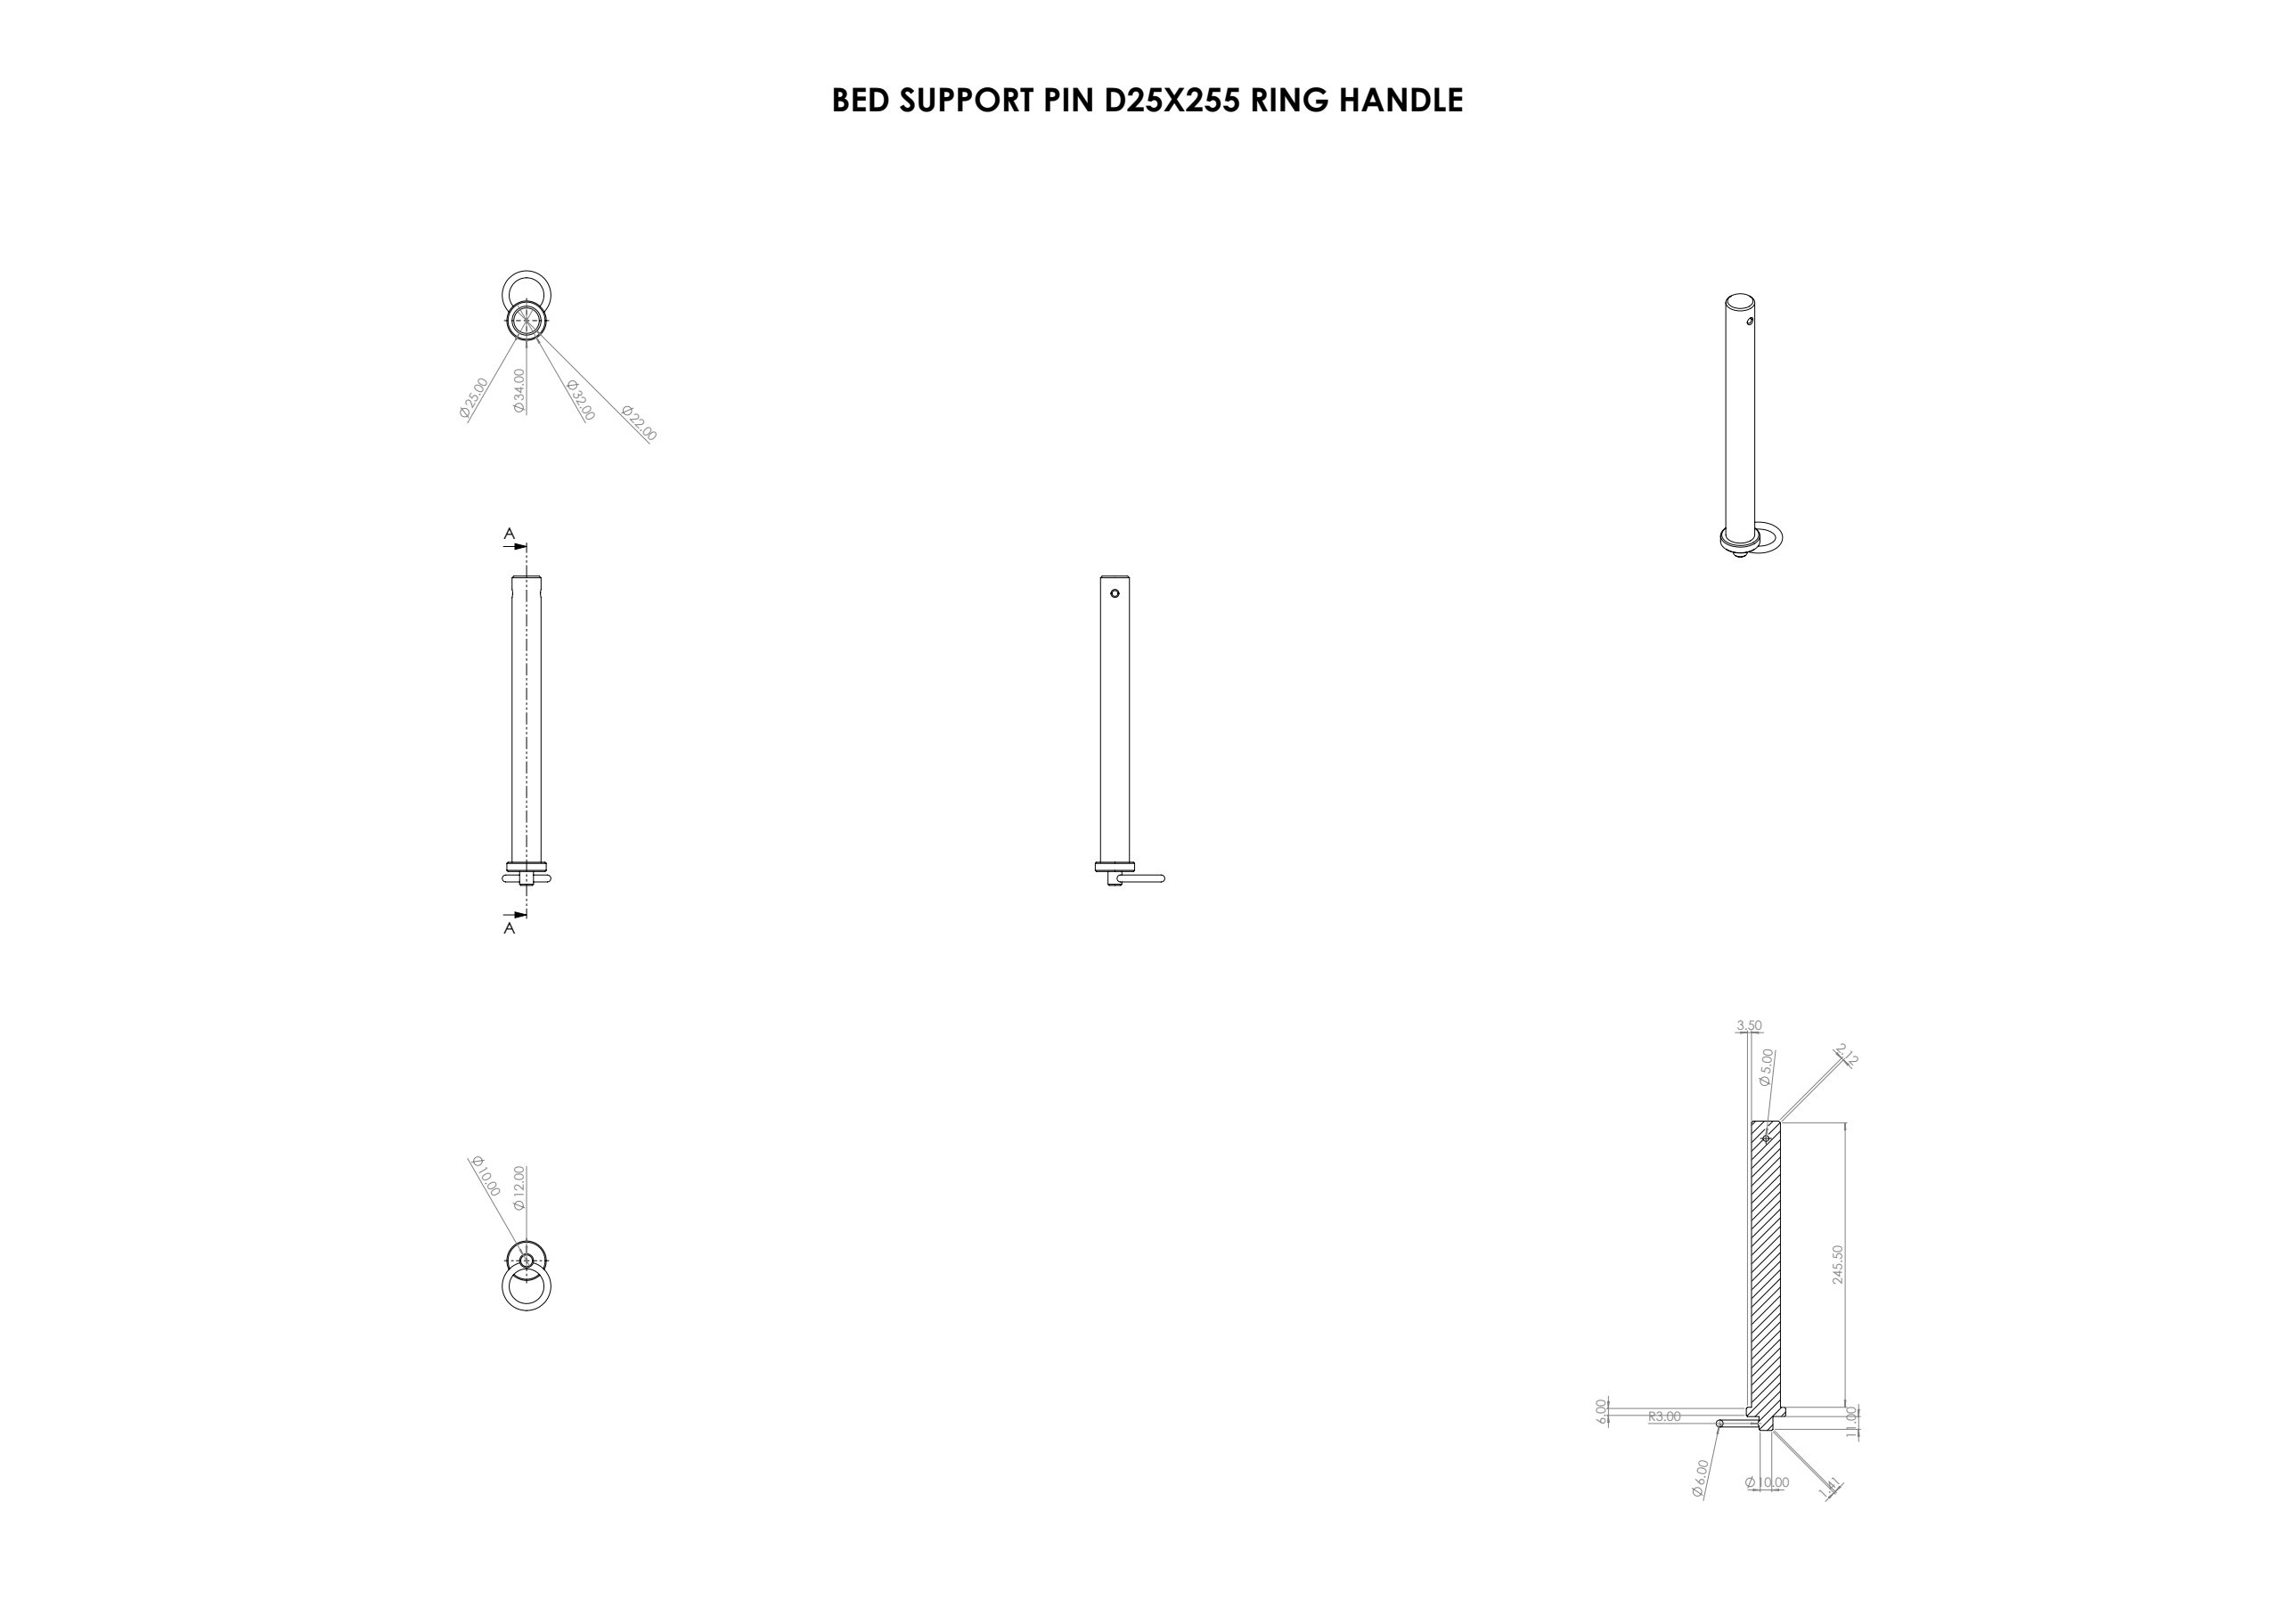
ISO-10303-21;
HEADER;
/* Generated by software containing ST-Developer
 * from STEP Tools, Inc. (www.steptools.com) 
 */

FILE_DESCRIPTION(
/* description */ (''),
/* implementation_level */ '2;1');

FILE_NAME(
/* name */ '05_Bed_Support_Pin_D25x255_Ring_Handle.step',
/* time_stamp */ '2026-10-20T10:03:03-07:00',
/* author */ (''),
/* organization */ (''),
/* preprocessor_version */ 'ST-DEVELOPER v20.2',
/* originating_system */ 'Autodesk Translation Framework v15.15.0.0',
/* authorisation */ '');

FILE_SCHEMA (('AUTOMOTIVE_DESIGN { 1 0 10303 214 3 1 1 }'));
ENDSEC;

DATA;
#10=MECHANICAL_DESIGN_GEOMETRIC_PRESENTATION_REPRESENTATION('',(#533),#71492);
#377=TOROIDAL_SURFACE('',#29987,1.8,0.299999999999997);
#390=SHAPE_REPRESENTATION_RELATIONSHIP('SRR','None',#71611,#409);
#409=ADVANCED_BREP_SHAPE_REPRESENTATION('',(#428),#71481);
#428=MANIFOLD_SOLID_BREP('Pin',#28467);
#533=STYLED_ITEM('',(#71887),#428);
#880=B_SPLINE_CURVE_WITH_KNOTS('',3,(#49263,#49264,#49265,#49266,#49267,
#49268,#49269,#49270,#49271,#49272,#49273,#49274,#49275,#49276,#49277,#49278,
#49279),.UNSPECIFIED.,.F.,.F.,(4,2,2,2,2,2,2,1,4),(0.,0.094448813972548,
0.188897627945096,0.283341149511147,0.377784671077197,0.472228192643248,
0.566671714209298,0.661120528181846,0.755569342154394),.UNSPECIFIED.);
#881=B_SPLINE_CURVE_WITH_KNOTS('',3,(#49280,#49281,#49282,#49283,#49284,
#49285,#49286,#49287,#49288,#49289,#49290,#49291,#49292,#49293,#49294,#49295,
#49296),.UNSPECIFIED.,.F.,.F.,(4,1,2,2,2,2,2,2,4),(0.755569342154394,0.850018156126942,
0.94446697009949,1.03891049166554,1.13335401323159,1.22779753479764,1.32224105636369,
1.41668987033624,1.51113868430879),.UNSPECIFIED.);
#882=B_SPLINE_CURVE_WITH_KNOTS('',3,(#49297,#49298,#49299,#49300,#49301,
#49302,#49303,#49304,#49305,#49306,#49307,#49308,#49309,#49310,#49311,#49312,
#49313,#49314,#49315,#49316,#49317,#49318,#49319,#49320,#49321,#49322,#49323,
#49324,#49325,#49326,#49327),.UNSPECIFIED.,.T.,.F.,(4,2,2,2,2,2,2,1,1,1,
2,2,2,2,2,2,4),(-1.51113868430879,-1.41668987033624,-1.32224105636369,-1.22779753479764,
-1.13335401323159,-1.03891049166554,-0.94446697009949,-0.850018156126942,
-0.755569342154394,-0.661120528181846,-0.566671714209298,-0.472228192643248,
-0.377784671077197,-0.283341149511147,-0.188897627945096,-0.094448813972548,
0.),.UNSPECIFIED.);
#883=B_SPLINE_CURVE_WITH_KNOTS('',3,(#49332,#49333,#49334,#49335,#49336,
#49337,#49338,#49339,#49340,#49341,#49342,#49343,#49344,#49345,#49346,#49347),
 .UNSPECIFIED.,.F.,.F.,(4,2,2,1,2,2,2,1,4),(0.,0.094448813972548,0.283341149511147,
0.330562910294172,0.377784671077197,0.472228192643248,0.566671714209298,
0.661120528181846,0.755569342154394),.UNSPECIFIED.);
#884=B_SPLINE_CURVE_WITH_KNOTS('',3,(#49348,#49349,#49350,#49351,#49352,
#49353,#49354,#49355,#49356,#49357,#49358,#49359,#49360,#49361,#49362,#49363,
#49364,#49365),.UNSPECIFIED.,.F.,.F.,(4,1,1,2,2,2,2,2,2,4),(0.755569342154394,
0.779181545647531,0.850018156126942,0.94446697009949,1.03891049166554,1.13335401323159,
1.22779753479764,1.32224105636369,1.41668987033624,1.51113868430879),
 .UNSPECIFIED.);
#885=B_SPLINE_CURVE_WITH_KNOTS('',3,(#49373,#49374,#49375,#49376,#49377,
#49378,#49379,#49380,#49381,#49382,#49383,#49384,#49385,#49386,#49387,#49388,
#49389,#49390,#49391,#49392,#49393,#49394,#49395,#49396,#49397,#49398,#49399,
#49400,#49401,#49402,#49403),.UNSPECIFIED.,.T.,.F.,(4,2,2,2,2,2,2,1,1,1,
1,2,2,2,1,2,2,4),(-1.51113868430879,-1.41668987033624,-1.32224105636369,
-1.22779753479764,-1.13335401323159,-1.03891049166554,-0.94446697009949,
-0.850018156126942,-0.779181545647531,-0.755569342154394,-0.661120528181846,
-0.566671714209298,-0.472228192643248,-0.377784671077197,-0.330562910294172,
-0.283341149511147,-0.094448813972548,0.),.UNSPECIFIED.);
#886=B_SPLINE_CURVE_WITH_KNOTS('',3,(#49535,#49536,#49537,#49538,#49539,
#49540,#49541,#49542),.UNSPECIFIED.,.F.,.F.,(4,2,2,4),(0.,0.128865571792524,
0.312353805988101,0.450725664145117),.UNSPECIFIED.);
#887=B_SPLINE_CURVE_WITH_KNOTS('',3,(#49544,#49545,#49546,#49547,#49548,
#49549,#49550,#49551,#49552,#49553,#49554,#49555,#49556,#49557,#49558,#49559,
#49560,#49561,#49562,#49563,#49564,#49565,#49566,#49567,#49568,#49569),
 .UNSPECIFIED.,.F.,.F.,(4,2,2,2,2,2,2,2,2,2,2,2,4),(3.03100409690103,3.10724965658915,
3.31962805616212,3.55816001091835,3.71946361604111,3.8667157448743,4.00577882547157,
4.14436012284324,4.2798687704017,4.40986006512752,4.53061941509967,4.63980546599939,
4.72630087619969),.UNSPECIFIED.);
#888=B_SPLINE_CURVE_WITH_KNOTS('',3,(#49570,#49571,#49572,#49573,#49574,
#49575,#49576,#49577,#49578,#49579,#49580,#49581,#49582,#49583,#49584,#49585,
#49586,#49587,#49588,#49589,#49590,#49591,#49592,#49593,#49594,#49595,#49596,
#49597,#49598,#49599,#49600,#49601),.UNSPECIFIED.,.F.,.F.,(4,2,2,2,2,2,
2,2,2,2,2,2,2,2,2,4),(0.450725664145117,0.504434541071938,0.741766796410238,
1.06081742489875,1.26362192220824,1.44561364264116,1.61660881920843,1.78645082881554,
1.9531313289519,2.11323423539159,2.26278985619793,2.3977184604128,2.53060287457306,
2.68742490157839,2.91311758246269,3.03100409690103),.UNSPECIFIED.);
#1458=B_SPLINE_SURFACE_WITH_KNOTS('',3,3,((#49135,#49136,#49137,#49138,
#49139,#49140,#49141,#49142,#49143,#49144,#49145,#49146,#49147,#49148,#49149,
#49150,#49151,#49152,#49153,#49154,#49155,#49156,#49157,#49158,#49159,#49160,
#49161,#49162,#49163,#49164,#49165),(#49166,#49167,#49168,#49169,#49170,
#49171,#49172,#49173,#49174,#49175,#49176,#49177,#49178,#49179,#49180,#49181,
#49182,#49183,#49184,#49185,#49186,#49187,#49188,#49189,#49190,#49191,#49192,
#49193,#49194,#49195,#49196),(#49197,#49198,#49199,#49200,#49201,#49202,
#49203,#49204,#49205,#49206,#49207,#49208,#49209,#49210,#49211,#49212,#49213,
#49214,#49215,#49216,#49217,#49218,#49219,#49220,#49221,#49222,#49223,#49224,
#49225,#49226,#49227),(#49228,#49229,#49230,#49231,#49232,#49233,#49234,
#49235,#49236,#49237,#49238,#49239,#49240,#49241,#49242,#49243,#49244,#49245,
#49246,#49247,#49248,#49249,#49250,#49251,#49252,#49253,#49254,#49255,#49256,
#49257,#49258)),.UNSPECIFIED.,.F.,.T.,.F.,(4,4),(4,2,2,2,2,2,2,1,1,1,2,
2,2,2,2,2,4),(0.,1.),(0.,0.094448813972548,0.188897627945096,0.283341149511147,
0.377784671077197,0.472228192643248,0.566671714209298,0.661120528181846,
0.755569342154394,0.850018156126942,0.94446697009949,1.03891049166554,1.13335401323159,
1.22779753479764,1.32224105636369,1.41668987033624,1.51113868430879),
 .UNSPECIFIED.);
#1459=B_SPLINE_SURFACE_WITH_KNOTS('',3,3,((#49404,#49405,#49406,#49407,
#49408,#49409,#49410,#49411,#49412,#49413,#49414,#49415,#49416,#49417,#49418,
#49419,#49420,#49421,#49422,#49423,#49424,#49425,#49426,#49427,#49428,#49429,
#49430,#49431,#49432,#49433,#49434),(#49435,#49436,#49437,#49438,#49439,
#49440,#49441,#49442,#49443,#49444,#49445,#49446,#49447,#49448,#49449,#49450,
#49451,#49452,#49453,#49454,#49455,#49456,#49457,#49458,#49459,#49460,#49461,
#49462,#49463,#49464,#49465),(#49466,#49467,#49468,#49469,#49470,#49471,
#49472,#49473,#49474,#49475,#49476,#49477,#49478,#49479,#49480,#49481,#49482,
#49483,#49484,#49485,#49486,#49487,#49488,#49489,#49490,#49491,#49492,#49493,
#49494,#49495,#49496),(#49497,#49498,#49499,#49500,#49501,#49502,#49503,
#49504,#49505,#49506,#49507,#49508,#49509,#49510,#49511,#49512,#49513,#49514,
#49515,#49516,#49517,#49518,#49519,#49520,#49521,#49522,#49523,#49524,#49525,
#49526,#49527)),.UNSPECIFIED.,.F.,.T.,.F.,(4,4),(4,2,2,1,2,2,2,1,1,1,1,
2,2,2,2,2,2,4),(0.,1.),(0.,0.094448813972548,0.283341149511147,0.330562910294172,
0.377784671077197,0.472228192643248,0.566671714209298,0.661120528181846,
0.755569342154394,0.779181545647531,0.850018156126942,0.94446697009949,
1.03891049166554,1.13335401323159,1.22779753479764,1.32224105636369,1.41668987033624,
1.51113868430879),.UNSPECIFIED.);
#1668=CYLINDRICAL_SURFACE('',#29983,0.25);
#1669=CYLINDRICAL_SURFACE('',#29984,1.25);
#1670=CYLINDRICAL_SURFACE('',#29990,0.599999999999994);
#1671=CYLINDRICAL_SURFACE('',#30000,1.7);
#1948=FACE_BOUND('',#5603,.T.);
#1949=FACE_BOUND('',#5604,.T.);
#1950=FACE_BOUND('',#5607,.T.);
#1951=FACE_BOUND('',#5612,.T.);
#1952=FACE_BOUND('',#5617,.T.);
#2465=CIRCLE('',#29985,1.25);
#2466=CIRCLE('',#29986,1.25);
#2467=CIRCLE('',#29988,0.299999999999997);
#2468=CIRCLE('',#29989,1.5);
#2469=CIRCLE('',#29991,0.599999999999994);
#2470=CIRCLE('',#29992,0.599999999999994);
#2471=CIRCLE('',#29994,0.5);
#2472=CIRCLE('',#29997,1.59999999999999);
#2473=CIRCLE('',#29999,1.7);
#2474=CIRCLE('',#30001,1.7);
#2475=CIRCLE('',#30003,1.59999999999999);
#2476=CIRCLE('',#30006,1.09999999999999);
#2861=CONICAL_SURFACE('',#29995,0.549999999999997,0.785398163397422);
#2862=CONICAL_SURFACE('',#29998,1.65000000000001,0.785398163397493);
#2863=CONICAL_SURFACE('',#30002,1.65000000000001,0.785398163397484);
#2864=CONICAL_SURFACE('',#30005,1.175,0.785398163397466);
#3946=FACE_OUTER_BOUND('',#5600,.T.);
#3947=FACE_OUTER_BOUND('',#5601,.T.);
#3948=FACE_OUTER_BOUND('',#5602,.T.);
#3949=FACE_OUTER_BOUND('',#5605,.T.);
#3950=FACE_OUTER_BOUND('',#5606,.T.);
#3951=FACE_OUTER_BOUND('',#5608,.T.);
#3952=FACE_OUTER_BOUND('',#5609,.T.);
#3953=FACE_OUTER_BOUND('',#5610,.T.);
#3954=FACE_OUTER_BOUND('',#5611,.T.);
#3955=FACE_OUTER_BOUND('',#5613,.T.);
#3956=FACE_OUTER_BOUND('',#5614,.T.);
#3957=FACE_OUTER_BOUND('',#5615,.T.);
#3958=FACE_OUTER_BOUND('',#5616,.T.);
#3959=FACE_OUTER_BOUND('',#5618,.T.);
#3960=FACE_OUTER_BOUND('',#5619,.T.);
#5600=EDGE_LOOP('',(#22975,#22976,#22977,#22978,#22979));
#5601=EDGE_LOOP('',(#22980,#22981,#22982,#22983,#22984,#22985));
#5602=EDGE_LOOP('',(#22986,#22987,#22988,#22989));
#5603=EDGE_LOOP('',(#22990));
#5604=EDGE_LOOP('',(#22991));
#5605=EDGE_LOOP('',(#22992,#22993,#22994,#22995,#22996));
#5606=EDGE_LOOP('',(#22997,#22998,#22999,#23000));
#5607=EDGE_LOOP('',(#23001,#23002,#23003));
#5608=EDGE_LOOP('',(#23004,#23005,#23006,#23007,#23008,#23009,#23010,#23011,
#23012));
#5609=EDGE_LOOP('',(#23013));
#5610=EDGE_LOOP('',(#23014,#23015,#23016,#23017));
#5611=EDGE_LOOP('',(#23018));
#5612=EDGE_LOOP('',(#23019));
#5613=EDGE_LOOP('',(#23020,#23021,#23022,#23023));
#5614=EDGE_LOOP('',(#23024,#23025,#23026,#23027));
#5615=EDGE_LOOP('',(#23028,#23029,#23030,#23031));
#5616=EDGE_LOOP('',(#23032));
#5617=EDGE_LOOP('',(#23033));
#5618=EDGE_LOOP('',(#23034,#23035,#23036,#23037));
#5619=EDGE_LOOP('',(#23038));
#7997=LINE('',#49261,#10485);
#7998=LINE('',#49330,#10486);
#7999=LINE('',#49370,#10487);
#8000=LINE('',#49528,#10488);
#8001=LINE('',#49605,#10489);
#8002=LINE('',#49607,#10490);
#8003=LINE('',#49613,#10491);
#8004=LINE('',#49620,#10492);
#8005=LINE('',#49624,#10493);
#8006=LINE('',#49628,#10494);
#8007=LINE('',#49633,#10495);
#10485=VECTOR('',#35140,1.);
#10486=VECTOR('',#35143,0.25);
#10487=VECTOR('',#35148,1.25);
#10488=VECTOR('',#35151,1.);
#10489=VECTOR('',#35162,0.599999999999994);
#10490=VECTOR('',#35163,0.599999999999994);
#10491=VECTOR('',#35172,0.549999999999997);
#10492=VECTOR('',#35181,1.65000000000001);
#10493=VECTOR('',#35186,1.7);
#10494=VECTOR('',#35191,1.65000000000001);
#10495=VECTOR('',#35198,1.175);
#12863=VERTEX_POINT('',#49259);
#12864=VERTEX_POINT('',#49260);
#12865=VERTEX_POINT('',#49262);
#12866=VERTEX_POINT('',#49329);
#12867=VERTEX_POINT('',#49331);
#12868=VERTEX_POINT('',#49367);
#12869=VERTEX_POINT('',#49369);
#12870=VERTEX_POINT('',#49372);
#12871=VERTEX_POINT('',#49530);
#12872=VERTEX_POINT('',#49533);
#12873=VERTEX_POINT('',#49534);
#12874=VERTEX_POINT('',#49543);
#12875=VERTEX_POINT('',#49603);
#12876=VERTEX_POINT('',#49606);
#12877=VERTEX_POINT('',#49610);
#12878=VERTEX_POINT('',#49615);
#12879=VERTEX_POINT('',#49618);
#12880=VERTEX_POINT('',#49622);
#12881=VERTEX_POINT('',#49626);
#12882=VERTEX_POINT('',#49631);
#16371=EDGE_CURVE('',#12863,#12864,#7997,.T.);
#16372=EDGE_CURVE('',#12864,#12865,#880,.T.);
#16373=EDGE_CURVE('',#12865,#12864,#881,.T.);
#16374=EDGE_CURVE('',#12863,#12863,#882,.T.);
#16375=EDGE_CURVE('',#12865,#12866,#7998,.T.);
#16376=EDGE_CURVE('',#12867,#12866,#883,.T.);
#16377=EDGE_CURVE('',#12866,#12867,#884,.T.);
#16378=EDGE_CURVE('',#12868,#12868,#2465,.T.);
#16379=EDGE_CURVE('',#12868,#12869,#7999,.T.);
#16380=EDGE_CURVE('',#12869,#12869,#2466,.T.);
#16381=EDGE_CURVE('',#12870,#12870,#885,.T.);
#16382=EDGE_CURVE('',#12870,#12867,#8000,.T.);
#16383=EDGE_CURVE('',#12871,#12871,#2467,.T.);
#16384=EDGE_CURVE('',#12871,#12871,#2468,.T.);
#16385=EDGE_CURVE('',#12872,#12873,#886,.T.);
#16386=EDGE_CURVE('',#12874,#12872,#887,.T.);
#16387=EDGE_CURVE('',#12873,#12874,#888,.T.);
#16388=EDGE_CURVE('',#12875,#12875,#2469,.T.);
#16389=EDGE_CURVE('',#12875,#12874,#8001,.T.);
#16390=EDGE_CURVE('',#12873,#12876,#8002,.T.);
#16391=EDGE_CURVE('',#12876,#12876,#2470,.T.);
#16392=EDGE_CURVE('',#12877,#12877,#2471,.T.);
#16393=EDGE_CURVE('',#12876,#12877,#8003,.T.);
#16394=EDGE_CURVE('',#12878,#12878,#2472,.T.);
#16395=EDGE_CURVE('',#12879,#12879,#2473,.T.);
#16396=EDGE_CURVE('',#12879,#12878,#8004,.T.);
#16397=EDGE_CURVE('',#12880,#12880,#2474,.T.);
#16398=EDGE_CURVE('',#12880,#12879,#8005,.T.);
#16399=EDGE_CURVE('',#12881,#12881,#2475,.T.);
#16400=EDGE_CURVE('',#12881,#12880,#8006,.T.);
#16401=EDGE_CURVE('',#12882,#12882,#2476,.T.);
#16402=EDGE_CURVE('',#12882,#12868,#8007,.T.);
#22975=ORIENTED_EDGE('',*,*,#16371,.T.);
#22976=ORIENTED_EDGE('',*,*,#16372,.T.);
#22977=ORIENTED_EDGE('',*,*,#16373,.T.);
#22978=ORIENTED_EDGE('',*,*,#16371,.F.);
#22979=ORIENTED_EDGE('',*,*,#16374,.T.);
#22980=ORIENTED_EDGE('',*,*,#16372,.F.);
#22981=ORIENTED_EDGE('',*,*,#16373,.F.);
#22982=ORIENTED_EDGE('',*,*,#16375,.T.);
#22983=ORIENTED_EDGE('',*,*,#16376,.F.);
#22984=ORIENTED_EDGE('',*,*,#16377,.F.);
#22985=ORIENTED_EDGE('',*,*,#16375,.F.);
#22986=ORIENTED_EDGE('',*,*,#16378,.F.);
#22987=ORIENTED_EDGE('',*,*,#16379,.T.);
#22988=ORIENTED_EDGE('',*,*,#16380,.T.);
#22989=ORIENTED_EDGE('',*,*,#16379,.F.);
#22990=ORIENTED_EDGE('',*,*,#16381,.F.);
#22991=ORIENTED_EDGE('',*,*,#16374,.F.);
#22992=ORIENTED_EDGE('',*,*,#16382,.T.);
#22993=ORIENTED_EDGE('',*,*,#16376,.T.);
#22994=ORIENTED_EDGE('',*,*,#16377,.T.);
#22995=ORIENTED_EDGE('',*,*,#16382,.F.);
#22996=ORIENTED_EDGE('',*,*,#16381,.T.);
#22997=ORIENTED_EDGE('',*,*,#16383,.F.);
#22998=ORIENTED_EDGE('',*,*,#16384,.T.);
#22999=ORIENTED_EDGE('',*,*,#16383,.T.);
#23000=ORIENTED_EDGE('',*,*,#16384,.F.);
#23001=ORIENTED_EDGE('',*,*,#16385,.F.);
#23002=ORIENTED_EDGE('',*,*,#16386,.F.);
#23003=ORIENTED_EDGE('',*,*,#16387,.F.);
#23004=ORIENTED_EDGE('',*,*,#16388,.F.);
#23005=ORIENTED_EDGE('',*,*,#16389,.T.);
#23006=ORIENTED_EDGE('',*,*,#16386,.T.);
#23007=ORIENTED_EDGE('',*,*,#16385,.T.);
#23008=ORIENTED_EDGE('',*,*,#16390,.T.);
#23009=ORIENTED_EDGE('',*,*,#16391,.T.);
#23010=ORIENTED_EDGE('',*,*,#16390,.F.);
#23011=ORIENTED_EDGE('',*,*,#16387,.T.);
#23012=ORIENTED_EDGE('',*,*,#16389,.F.);
#23013=ORIENTED_EDGE('',*,*,#16392,.F.);
#23014=ORIENTED_EDGE('',*,*,#16391,.F.);
#23015=ORIENTED_EDGE('',*,*,#16393,.T.);
#23016=ORIENTED_EDGE('',*,*,#16392,.T.);
#23017=ORIENTED_EDGE('',*,*,#16393,.F.);
#23018=ORIENTED_EDGE('',*,*,#16394,.F.);
#23019=ORIENTED_EDGE('',*,*,#16388,.T.);
#23020=ORIENTED_EDGE('',*,*,#16395,.F.);
#23021=ORIENTED_EDGE('',*,*,#16396,.T.);
#23022=ORIENTED_EDGE('',*,*,#16394,.T.);
#23023=ORIENTED_EDGE('',*,*,#16396,.F.);
#23024=ORIENTED_EDGE('',*,*,#16397,.F.);
#23025=ORIENTED_EDGE('',*,*,#16398,.T.);
#23026=ORIENTED_EDGE('',*,*,#16395,.T.);
#23027=ORIENTED_EDGE('',*,*,#16398,.F.);
#23028=ORIENTED_EDGE('',*,*,#16399,.F.);
#23029=ORIENTED_EDGE('',*,*,#16400,.T.);
#23030=ORIENTED_EDGE('',*,*,#16397,.T.);
#23031=ORIENTED_EDGE('',*,*,#16400,.F.);
#23032=ORIENTED_EDGE('',*,*,#16399,.T.);
#23033=ORIENTED_EDGE('',*,*,#16380,.F.);
#23034=ORIENTED_EDGE('',*,*,#16401,.F.);
#23035=ORIENTED_EDGE('',*,*,#16402,.T.);
#23036=ORIENTED_EDGE('',*,*,#16378,.T.);
#23037=ORIENTED_EDGE('',*,*,#16402,.F.);
#23038=ORIENTED_EDGE('',*,*,#16401,.T.);
#26669=PLANE('',#29993);
#26670=PLANE('',#29996);
#26671=PLANE('',#30004);
#26672=PLANE('',#30007);
#27854=ADVANCED_FACE('',(#3946),#1458,.T.);
#27855=ADVANCED_FACE('',(#3947),#1668,.F.);
#27856=ADVANCED_FACE('',(#3948,#1948,#1949),#1669,.T.);
#27857=ADVANCED_FACE('',(#3949),#1459,.T.);
#27858=ADVANCED_FACE('',(#3950,#1950),#377,.T.);
#27859=ADVANCED_FACE('',(#3951),#1670,.T.);
#27860=ADVANCED_FACE('',(#3952),#26669,.T.);
#27861=ADVANCED_FACE('',(#3953),#2861,.T.);
#27862=ADVANCED_FACE('',(#3954,#1951),#26670,.T.);
#27863=ADVANCED_FACE('',(#3955),#2862,.T.);
#27864=ADVANCED_FACE('',(#3956),#1671,.T.);
#27865=ADVANCED_FACE('',(#3957),#2863,.T.);
#27866=ADVANCED_FACE('',(#3958,#1952),#26671,.T.);
#27867=ADVANCED_FACE('',(#3959),#2864,.T.);
#27868=ADVANCED_FACE('',(#3960),#26672,.T.);
#28467=CLOSED_SHELL('',(#27854,#27855,#27856,#27857,#27858,#27859,#27860,
#27861,#27862,#27863,#27864,#27865,#27866,#27867,#27868));
#29982=AXIS2_PLACEMENT_3D('',#49134,#35138,#35139);
#29983=AXIS2_PLACEMENT_3D('',#49328,#35141,#35142);
#29984=AXIS2_PLACEMENT_3D('',#49366,#35144,#35145);
#29985=AXIS2_PLACEMENT_3D('',#49368,#35146,#35147);
#29986=AXIS2_PLACEMENT_3D('',#49371,#35149,#35150);
#29987=AXIS2_PLACEMENT_3D('',#49529,#35152,#35153);
#29988=AXIS2_PLACEMENT_3D('',#49531,#35154,#35155);
#29989=AXIS2_PLACEMENT_3D('',#49532,#35156,#35157);
#29990=AXIS2_PLACEMENT_3D('',#49602,#35158,#35159);
#29991=AXIS2_PLACEMENT_3D('',#49604,#35160,#35161);
#29992=AXIS2_PLACEMENT_3D('',#49608,#35164,#35165);
#29993=AXIS2_PLACEMENT_3D('',#49609,#35166,#35167);
#29994=AXIS2_PLACEMENT_3D('',#49611,#35168,#35169);
#29995=AXIS2_PLACEMENT_3D('',#49612,#35170,#35171);
#29996=AXIS2_PLACEMENT_3D('',#49614,#35173,#35174);
#29997=AXIS2_PLACEMENT_3D('',#49616,#35175,#35176);
#29998=AXIS2_PLACEMENT_3D('',#49617,#35177,#35178);
#29999=AXIS2_PLACEMENT_3D('',#49619,#35179,#35180);
#30000=AXIS2_PLACEMENT_3D('',#49621,#35182,#35183);
#30001=AXIS2_PLACEMENT_3D('',#49623,#35184,#35185);
#30002=AXIS2_PLACEMENT_3D('',#49625,#35187,#35188);
#30003=AXIS2_PLACEMENT_3D('',#49627,#35189,#35190);
#30004=AXIS2_PLACEMENT_3D('',#49629,#35192,#35193);
#30005=AXIS2_PLACEMENT_3D('',#49630,#35194,#35195);
#30006=AXIS2_PLACEMENT_3D('',#49632,#35196,#35197);
#30007=AXIS2_PLACEMENT_3D('',#49634,#35199,#35200);
#35138=DIRECTION('axis',(0.,0.,1.));
#35139=DIRECTION('refdir',(1.,0.,0.));
#35140=DIRECTION('',(0.616833943686132,1.43989874226525E-14,0.787093314618168));
#35141=DIRECTION('center_axis',(1.,0.,0.));
#35142=DIRECTION('ref_axis',(0.,0.,-1.));
#35143=DIRECTION('',(1.,0.,0.));
#35144=DIRECTION('center_axis',(0.,1.,0.));
#35145=DIRECTION('ref_axis',(0.,0.,1.));
#35146=DIRECTION('center_axis',(0.,1.,0.));
#35147=DIRECTION('ref_axis',(1.,0.,0.));
#35148=DIRECTION('',(0.,-1.,0.));
#35149=DIRECTION('center_axis',(0.,1.,0.));
#35150=DIRECTION('ref_axis',(1.,0.,0.));
#35151=DIRECTION('',(-0.616833943686132,0.,0.787093314618168));
#35152=DIRECTION('center_axis',(0.,1.,0.));
#35153=DIRECTION('ref_axis',(0.,0.,1.));
#35154=DIRECTION('center_axis',(-1.,0.,0.));
#35155=DIRECTION('ref_axis',(0.,0.,-1.));
#35156=DIRECTION('center_axis',(0.,-1.,0.));
#35157=DIRECTION('ref_axis',(0.,0.,1.));
#35158=DIRECTION('center_axis',(0.,1.,0.));
#35159=DIRECTION('ref_axis',(0.,0.,1.));
#35160=DIRECTION('center_axis',(0.,1.,0.));
#35161=DIRECTION('ref_axis',(0.,0.,1.));
#35162=DIRECTION('',(0.,-1.,0.));
#35163=DIRECTION('',(0.,-1.,0.));
#35164=DIRECTION('center_axis',(0.,1.,0.));
#35165=DIRECTION('ref_axis',(1.,0.,0.));
#35166=DIRECTION('center_axis',(0.,-1.,0.));
#35167=DIRECTION('ref_axis',(0.,0.,-1.));
#35168=DIRECTION('center_axis',(0.,1.,0.));
#35169=DIRECTION('ref_axis',(1.,0.,0.));
#35170=DIRECTION('center_axis',(0.,1.,0.));
#35171=DIRECTION('ref_axis',(0.,0.,1.));
#35172=DIRECTION('',(8.6595605623547E-17,-0.707106781186566,0.707106781186529));
#35173=DIRECTION('center_axis',(0.,-1.,0.));
#35174=DIRECTION('ref_axis',(0.,0.,-1.));
#35175=DIRECTION('center_axis',(0.,1.,0.));
#35176=DIRECTION('ref_axis',(1.,0.,0.));
#35177=DIRECTION('center_axis',(0.,1.,0.));
#35178=DIRECTION('ref_axis',(0.,0.,1.));
#35179=DIRECTION('center_axis',(0.,1.,0.));
#35180=DIRECTION('ref_axis',(1.,0.,0.));
#35181=DIRECTION('',(8.65956056235532E-17,-0.707106781186516,0.707106781186579));
#35182=DIRECTION('center_axis',(0.,1.,0.));
#35183=DIRECTION('ref_axis',(0.,0.,1.));
#35184=DIRECTION('center_axis',(0.,1.,0.));
#35185=DIRECTION('ref_axis',(1.,0.,0.));
#35186=DIRECTION('',(0.,-1.,0.));
#35187=DIRECTION('center_axis',(0.,-1.,0.));
#35188=DIRECTION('ref_axis',(0.,0.,1.));
#35189=DIRECTION('center_axis',(0.,1.,0.));
#35190=DIRECTION('ref_axis',(1.,0.,0.));
#35191=DIRECTION('',(-8.65956056235524E-17,-0.707106781186522,-0.707106781186573));
#35192=DIRECTION('center_axis',(0.,1.,0.));
#35193=DIRECTION('ref_axis',(0.,0.,1.));
#35194=DIRECTION('center_axis',(0.,-1.,0.));
#35195=DIRECTION('ref_axis',(0.,0.,1.));
#35196=DIRECTION('center_axis',(0.,1.,0.));
#35197=DIRECTION('ref_axis',(1.,0.,0.));
#35198=DIRECTION('',(-8.65956056235509E-17,-0.707106781186535,-0.70710678118656));
#35199=DIRECTION('center_axis',(0.,1.,0.));
#35200=DIRECTION('ref_axis',(0.,0.,1.));
#49134=CARTESIAN_POINT('',(0.,0.,0.));
#49135=CARTESIAN_POINT('Ctrl Pts',(28.7991583057917,11.,74.402898825339));
#49136=CARTESIAN_POINT('Ctrl Pts',(28.7991583057917,11.0443255072037,74.402898825339));
#49137=CARTESIAN_POINT('Ctrl Pts',(28.7965453592084,11.0915510411579,74.4116063134345));
#49138=CARTESIAN_POINT('Ctrl Pts',(28.7871669871617,11.1779078402817,74.4468238161368));
#49139=CARTESIAN_POINT('Ctrl Pts',(28.7806043669257,11.2170846527409,74.4732883033298));
#49140=CARTESIAN_POINT('Ctrl Pts',(28.7683045654192,11.2788962751735,74.5344620266402));
#49141=CARTESIAN_POINT('Ctrl Pts',(28.7617930434695,11.3057060685816,74.5732868944695));
#49142=CARTESIAN_POINT('Ctrl Pts',(28.7525231854577,11.3414465815878,74.65904064169));
#49143=CARTESIAN_POINT('Ctrl Pts',(28.7499823739105,11.3502679248349,74.7059347785805));
#49144=CARTESIAN_POINT('Ctrl Pts',(28.7499717367413,11.3503212800739,74.7941254313177));
#49145=CARTESIAN_POINT('Ctrl Pts',(28.7525477553864,11.3414466364947,74.8410052800481));
#49146=CARTESIAN_POINT('Ctrl Pts',(28.7618133828337,11.3058394721478,74.9267618361903));
#49147=CARTESIAN_POINT('Ctrl Pts',(28.7683297787118,11.2789656668451,74.9656153280843));
#49148=CARTESIAN_POINT('Ctrl Pts',(28.7806136472154,11.2174765285995,75.0267085651774));
#49149=CARTESIAN_POINT('Ctrl Pts',(28.7938779355307,11.137485266407,75.079826557824));
#49150=CARTESIAN_POINT('Ctrl Pts',(28.8019055096204,11.,75.1059958179575));
#49151=CARTESIAN_POINT('Ctrl Pts',(28.7938779355307,10.8625147335932,75.079826557824));
#49152=CARTESIAN_POINT('Ctrl Pts',(28.7806136472154,10.7825234714004,75.0267085651771));
#49153=CARTESIAN_POINT('Ctrl Pts',(28.7683297787118,10.7210343331551,74.9656153280842));
#49154=CARTESIAN_POINT('Ctrl Pts',(28.7618133828337,10.6941605278523,74.9267618361901));
#49155=CARTESIAN_POINT('Ctrl Pts',(28.7525477553864,10.6585533635054,74.8410052800478));
#49156=CARTESIAN_POINT('Ctrl Pts',(28.7499717367413,10.6496787199262,74.7941254313175));
#49157=CARTESIAN_POINT('Ctrl Pts',(28.7499823739105,10.6497320751652,74.7059347785801));
#49158=CARTESIAN_POINT('Ctrl Pts',(28.7525231854577,10.6585534184123,74.6590406416897));
#49159=CARTESIAN_POINT('Ctrl Pts',(28.7617930434695,10.6942939314186,74.5732868944692));
#49160=CARTESIAN_POINT('Ctrl Pts',(28.7683045654192,10.7211037248264,74.5344620266403));
#49161=CARTESIAN_POINT('Ctrl Pts',(28.7806043669256,10.7829153472589,74.4732883033299));
#49162=CARTESIAN_POINT('Ctrl Pts',(28.7871669871616,10.8220921597181,74.4468238161368));
#49163=CARTESIAN_POINT('Ctrl Pts',(28.7965453592083,10.9084489588421,74.4116063134345));
#49164=CARTESIAN_POINT('Ctrl Pts',(28.7991583057917,10.9556744927962,74.402898825339));
#49165=CARTESIAN_POINT('Ctrl Pts',(28.7991583057917,11.,74.402898825339));
#49166=CARTESIAN_POINT('Ctrl Pts',(28.8245239133973,11.,74.4352658835594));
#49167=CARTESIAN_POINT('Ctrl Pts',(28.8245139996716,11.0409058476698,74.4352690808426));
#49168=CARTESIAN_POINT('Ctrl Pts',(28.8222946915156,11.0844693260521,74.4435587606527));
#49169=CARTESIAN_POINT('Ctrl Pts',(28.8143446526051,11.1634798118501,74.4766846891437));
#49170=CARTESIAN_POINT('Ctrl Pts',(28.8088018057836,11.1989487338351,74.5013491133979));
#49171=CARTESIAN_POINT('Ctrl Pts',(28.7984971202627,11.2543047022451,74.5574809291687));
#49172=CARTESIAN_POINT('Ctrl Pts',(28.7930705898665,11.277994263562,74.5926796862592));
#49173=CARTESIAN_POINT('Ctrl Pts',(28.7854083939203,11.3092896913271,74.6694190769384));
#49174=CARTESIAN_POINT('Ctrl Pts',(28.783317023756,11.316933318266,74.7109865811412));
#49175=CARTESIAN_POINT('Ctrl Pts',(28.7833092717601,11.3169759220082,74.789072841938));
#49176=CARTESIAN_POINT('Ctrl Pts',(28.7854300007706,11.3093021925761,74.8306284308288));
#49177=CARTESIAN_POINT('Ctrl Pts',(28.7930936893998,11.2781129419873,74.9073660164418));
#49178=CARTESIAN_POINT('Ctrl Pts',(28.7985190764957,11.2543992363159,74.9426040045736));
#49179=CARTESIAN_POINT('Ctrl Pts',(28.8088155168561,11.1992993473659,74.998632839126));
#49180=CARTESIAN_POINT('Ctrl Pts',(28.8200190370477,11.1268998693587,75.0482404349203));
#49181=CARTESIAN_POINT('Ctrl Pts',(28.8268763497815,11.,75.0732472458756));
#49182=CARTESIAN_POINT('Ctrl Pts',(28.8200190370477,10.8731001306415,75.0482404349203));
#49183=CARTESIAN_POINT('Ctrl Pts',(28.8088155168561,10.8007006526339,74.9986328391256));
#49184=CARTESIAN_POINT('Ctrl Pts',(28.7985190764957,10.7456007636843,74.9426040045735));
#49185=CARTESIAN_POINT('Ctrl Pts',(28.7930936893998,10.7218870580128,74.9073660164416));
#49186=CARTESIAN_POINT('Ctrl Pts',(28.7854300007706,10.690697807424,74.8306284308285));
#49187=CARTESIAN_POINT('Ctrl Pts',(28.78330927176,10.6830240779919,74.7890728419378));
#49188=CARTESIAN_POINT('Ctrl Pts',(28.783317023756,10.6830666817342,74.7109865811408));
#49189=CARTESIAN_POINT('Ctrl Pts',(28.7854083939203,10.6907103086731,74.669419076938));
#49190=CARTESIAN_POINT('Ctrl Pts',(28.7930705898666,10.7220057364382,74.5926796862589));
#49191=CARTESIAN_POINT('Ctrl Pts',(28.7984971202626,10.7456952977549,74.5574809291687));
#49192=CARTESIAN_POINT('Ctrl Pts',(28.8088018057835,10.8010512661648,74.501349113398));
#49193=CARTESIAN_POINT('Ctrl Pts',(28.8143446526051,10.8365201881497,74.4766846891437));
#49194=CARTESIAN_POINT('Ctrl Pts',(28.8222946915156,10.9155306739479,74.4435587606527));
#49195=CARTESIAN_POINT('Ctrl Pts',(28.8245139996716,10.9590941523302,74.4352690808426));
#49196=CARTESIAN_POINT('Ctrl Pts',(28.8245239133973,11.,74.4352658835594));
#49197=CARTESIAN_POINT('Ctrl Pts',(28.8498895210029,11.,74.4676329417797));
#49198=CARTESIAN_POINT('Ctrl Pts',(28.8498994347286,11.0374731686475,74.4676297444964));
#49199=CARTESIAN_POINT('Ctrl Pts',(28.8480500789078,11.0773718356336,74.4755355640341));
#49200=CARTESIAN_POINT('Ctrl Pts',(28.8415279162029,11.1490230557141,74.5065180699672));
#49201=CARTESIAN_POINT('Ctrl Pts',(28.8370145392765,11.1807553920361,74.5294168541035));
#49202=CARTESIAN_POINT('Ctrl Pts',(28.8286875791424,11.2296820491551,74.5804873246879));
#49203=CARTESIAN_POINT('Ctrl Pts',(28.82436943821,11.2501911813549,74.6120535237142));
#49204=CARTESIAN_POINT('Ctrl Pts',(28.8182862167288,11.2770897699908,74.6798098456223));
#49205=CARTESIAN_POINT('Ctrl Pts',(28.8166559433367,11.2835149969489,74.7160141451695));
#49206=CARTESIAN_POINT('Ctrl Pts',(28.8166480659251,11.2835588407745,74.7840389985826));
#49207=CARTESIAN_POINT('Ctrl Pts',(28.8183009558858,11.2770859558961,74.8202442285893));
#49208=CARTESIAN_POINT('Ctrl Pts',(28.824374236808,11.25031714301,74.8879969147892));
#49209=CARTESIAN_POINT('Ctrl Pts',(28.8287019700868,11.229715550308,74.9195760683006));
#49210=CARTESIAN_POINT('Ctrl Pts',(28.8370133377376,11.1810854764448,74.9706146871361));
#49211=CARTESIAN_POINT('Ctrl Pts',(28.8461514336814,11.1161862398084,75.0165933605779));
#49212=CARTESIAN_POINT('Ctrl Pts',(28.85182326022,11.,75.0405083037254));
#49213=CARTESIAN_POINT('Ctrl Pts',(28.8461514336813,10.8838137601915,75.0165933605779));
#49214=CARTESIAN_POINT('Ctrl Pts',(28.8370133377375,10.8189145235551,74.970614687136));
#49215=CARTESIAN_POINT('Ctrl Pts',(28.8287019700867,10.7702844496919,74.9195760683005));
#49216=CARTESIAN_POINT('Ctrl Pts',(28.824374236808,10.7496828569899,74.8879969147891));
#49217=CARTESIAN_POINT('Ctrl Pts',(28.8183009558857,10.7229140441039,74.8202442285892));
#49218=CARTESIAN_POINT('Ctrl Pts',(28.816648065925,10.7164411592254,74.7840389985825));
#49219=CARTESIAN_POINT('Ctrl Pts',(28.8166559433366,10.716485003051,74.7160141451694));
#49220=CARTESIAN_POINT('Ctrl Pts',(28.8182862167287,10.7229102300091,74.6798098456222));
#49221=CARTESIAN_POINT('Ctrl Pts',(28.82436943821,10.749808818645,74.6120535237141));
#49222=CARTESIAN_POINT('Ctrl Pts',(28.8286875791424,10.7703179508449,74.5804873246878));
#49223=CARTESIAN_POINT('Ctrl Pts',(28.8370145392765,10.8192446079639,74.5294168541034));
#49224=CARTESIAN_POINT('Ctrl Pts',(28.8415279162029,10.8509769442859,74.5065180699671));
#49225=CARTESIAN_POINT('Ctrl Pts',(28.8480500789077,10.9226281643664,74.475535564034));
#49226=CARTESIAN_POINT('Ctrl Pts',(28.8498994347286,10.9625268313525,74.4676297444964));
#49227=CARTESIAN_POINT('Ctrl Pts',(28.8498895210029,11.,74.4676329417797));
#49228=CARTESIAN_POINT('Ctrl Pts',(28.8752551286084,11.,74.5));
#49229=CARTESIAN_POINT('Ctrl Pts',(28.8752551286084,11.0340535091136,74.5));
#49230=CARTESIAN_POINT('Ctrl Pts',(28.873799411215,11.0702901205278,74.5074880112523));
#49231=CARTESIAN_POINT('Ctrl Pts',(28.8687055816464,11.1345950272825,74.5363789429741));
#49232=CARTESIAN_POINT('Ctrl Pts',(28.8652119781344,11.1626194731303,74.5574776641716));
#49233=CARTESIAN_POINT('Ctrl Pts',(28.8588801339858,11.2050904762266,74.6035062272164));
#49234=CARTESIAN_POINT('Ctrl Pts',(28.8556469846071,11.2224793763353,74.6314463155039));
#49235=CARTESIAN_POINT('Ctrl Pts',(28.8511714251914,11.2449328797301,74.6901882808707));
#49236=CARTESIAN_POINT('Ctrl Pts',(28.8499905931822,11.2501803903799,74.7210659477303));
#49237=CARTESIAN_POINT('Ctrl Pts',(28.8499856009438,11.2502134827088,74.778986409203));
#49238=CARTESIAN_POINT('Ctrl Pts',(28.85118320127,11.2449415119774,74.80986737937));
#49239=CARTESIAN_POINT('Ctrl Pts',(28.8556545433741,11.2225906128495,74.8686010950407));
#49240=CARTESIAN_POINT('Ctrl Pts',(28.8588912678706,11.2051491197789,74.8965647447899));
#49241=CARTESIAN_POINT('Ctrl Pts',(28.8652152073783,11.1629082952113,74.9425389610847));
#49242=CARTESIAN_POINT('Ctrl Pts',(28.8722925351983,11.1056008427601,74.9850072376742));
#49243=CARTESIAN_POINT('Ctrl Pts',(28.8767941003811,11.,75.0077597316435));
#49244=CARTESIAN_POINT('Ctrl Pts',(28.8722925351983,10.8943991572398,74.9850072376742));
#49245=CARTESIAN_POINT('Ctrl Pts',(28.8652152073782,10.8370917047886,74.9425389610846));
#49246=CARTESIAN_POINT('Ctrl Pts',(28.8588912678706,10.794850880221,74.8965647447899));
#49247=CARTESIAN_POINT('Ctrl Pts',(28.8556545433741,10.7774093871504,74.8686010950406));
#49248=CARTESIAN_POINT('Ctrl Pts',(28.8511832012699,10.7550584880225,74.8098673793699));
#49249=CARTESIAN_POINT('Ctrl Pts',(28.8499856009438,10.7497865172911,74.7789864092028));
#49250=CARTESIAN_POINT('Ctrl Pts',(28.8499905931821,10.74981960962,74.7210659477302));
#49251=CARTESIAN_POINT('Ctrl Pts',(28.8511714251913,10.7550671202698,74.6901882808706));
#49252=CARTESIAN_POINT('Ctrl Pts',(28.8556469846071,10.7775206236646,74.6314463155038));
#49253=CARTESIAN_POINT('Ctrl Pts',(28.8588801339858,10.7949095237734,74.6035062272163));
#49254=CARTESIAN_POINT('Ctrl Pts',(28.8652119781344,10.8373805268697,74.5574776641715));
#49255=CARTESIAN_POINT('Ctrl Pts',(28.8687055816464,10.8654049727175,74.536378942974));
#49256=CARTESIAN_POINT('Ctrl Pts',(28.873799411215,10.9297098794722,74.5074880112522));
#49257=CARTESIAN_POINT('Ctrl Pts',(28.8752551286084,10.9659464908864,74.5));
#49258=CARTESIAN_POINT('Ctrl Pts',(28.8752551286084,11.,74.5));
#49259=CARTESIAN_POINT('',(28.7991583057917,11.,74.402898825339));
#49260=CARTESIAN_POINT('',(28.8752551286084,11.,74.5));
#49261=CARTESIAN_POINT('',(28.7991583057917,11.,74.402898825339));
#49262=CARTESIAN_POINT('',(28.8752935786535,11.,75.000175566987));
#49263=CARTESIAN_POINT('Ctrl Pts',(28.8752551286084,11.,74.5));
#49264=CARTESIAN_POINT('Ctrl Pts',(28.8752551286084,11.0340535091136,74.5));
#49265=CARTESIAN_POINT('Ctrl Pts',(28.873799411215,11.0702901205278,74.5074880112523));
#49266=CARTESIAN_POINT('Ctrl Pts',(28.8687055816464,11.1345950272825,74.5363789429741));
#49267=CARTESIAN_POINT('Ctrl Pts',(28.8652119781344,11.1626194731303,74.5574776641716));
#49268=CARTESIAN_POINT('Ctrl Pts',(28.8588801339858,11.2050904762266,74.6035062272164));
#49269=CARTESIAN_POINT('Ctrl Pts',(28.8556469846071,11.2224793763353,74.6314463155039));
#49270=CARTESIAN_POINT('Ctrl Pts',(28.8511714251914,11.2449328797301,74.6901882808707));
#49271=CARTESIAN_POINT('Ctrl Pts',(28.8499905931822,11.2501803903799,74.7210659477303));
#49272=CARTESIAN_POINT('Ctrl Pts',(28.8499856009438,11.2502134827088,74.778986409203));
#49273=CARTESIAN_POINT('Ctrl Pts',(28.85118320127,11.2449415119774,74.80986737937));
#49274=CARTESIAN_POINT('Ctrl Pts',(28.8556545433741,11.2225906128495,74.8686010950407));
#49275=CARTESIAN_POINT('Ctrl Pts',(28.8588912678706,11.2051491197789,74.8965647447899));
#49276=CARTESIAN_POINT('Ctrl Pts',(28.8652152073783,11.1629082952113,74.9425389610847));
#49277=CARTESIAN_POINT('Ctrl Pts',(28.8722925351983,11.1056008427601,74.9850072376742));
#49278=CARTESIAN_POINT('Ctrl Pts',(28.8752935786535,11.03520028092,75.000175566987));
#49279=CARTESIAN_POINT('Ctrl Pts',(28.8752935786535,11.,75.000175566987));
#49280=CARTESIAN_POINT('Ctrl Pts',(28.8752935786535,11.,75.000175566987));
#49281=CARTESIAN_POINT('Ctrl Pts',(28.8752935786535,10.9647997190799,75.000175566987));
#49282=CARTESIAN_POINT('Ctrl Pts',(28.8722925351983,10.8943991572398,74.9850072376742));
#49283=CARTESIAN_POINT('Ctrl Pts',(28.8652152073782,10.8370917047886,74.9425389610846));
#49284=CARTESIAN_POINT('Ctrl Pts',(28.8588912678706,10.794850880221,74.8965647447899));
#49285=CARTESIAN_POINT('Ctrl Pts',(28.8556545433741,10.7774093871504,74.8686010950406));
#49286=CARTESIAN_POINT('Ctrl Pts',(28.8511832012699,10.7550584880225,74.8098673793699));
#49287=CARTESIAN_POINT('Ctrl Pts',(28.8499856009438,10.7497865172911,74.7789864092028));
#49288=CARTESIAN_POINT('Ctrl Pts',(28.8499905931821,10.74981960962,74.7210659477302));
#49289=CARTESIAN_POINT('Ctrl Pts',(28.8511714251913,10.7550671202698,74.6901882808706));
#49290=CARTESIAN_POINT('Ctrl Pts',(28.8556469846071,10.7775206236646,74.6314463155038));
#49291=CARTESIAN_POINT('Ctrl Pts',(28.8588801339858,10.7949095237734,74.6035062272163));
#49292=CARTESIAN_POINT('Ctrl Pts',(28.8652119781344,10.8373805268697,74.5574776641715));
#49293=CARTESIAN_POINT('Ctrl Pts',(28.8687055816464,10.8654049727175,74.536378942974));
#49294=CARTESIAN_POINT('Ctrl Pts',(28.873799411215,10.9297098794722,74.5074880112522));
#49295=CARTESIAN_POINT('Ctrl Pts',(28.8752551286084,10.9659464908864,74.5));
#49296=CARTESIAN_POINT('Ctrl Pts',(28.8752551286084,11.,74.5));
#49297=CARTESIAN_POINT('Ctrl Pts',(28.7991583057917,11.,74.402898825339));
#49298=CARTESIAN_POINT('Ctrl Pts',(28.7991583057917,10.9556744927962,74.402898825339));
#49299=CARTESIAN_POINT('Ctrl Pts',(28.7965453592083,10.9084489588421,74.4116063134345));
#49300=CARTESIAN_POINT('Ctrl Pts',(28.7871669871616,10.8220921597181,74.4468238161368));
#49301=CARTESIAN_POINT('Ctrl Pts',(28.7806043669256,10.7829153472589,74.4732883033299));
#49302=CARTESIAN_POINT('Ctrl Pts',(28.7683045654192,10.7211037248264,74.5344620266403));
#49303=CARTESIAN_POINT('Ctrl Pts',(28.7617930434695,10.6942939314186,74.5732868944692));
#49304=CARTESIAN_POINT('Ctrl Pts',(28.7525231854577,10.6585534184123,74.6590406416897));
#49305=CARTESIAN_POINT('Ctrl Pts',(28.7499823739105,10.6497320751652,74.7059347785801));
#49306=CARTESIAN_POINT('Ctrl Pts',(28.7499717367413,10.6496787199262,74.7941254313175));
#49307=CARTESIAN_POINT('Ctrl Pts',(28.7525477553864,10.6585533635054,74.8410052800478));
#49308=CARTESIAN_POINT('Ctrl Pts',(28.7618133828337,10.6941605278523,74.9267618361901));
#49309=CARTESIAN_POINT('Ctrl Pts',(28.7683297787118,10.7210343331551,74.9656153280842));
#49310=CARTESIAN_POINT('Ctrl Pts',(28.7806136472154,10.7825234714004,75.0267085651771));
#49311=CARTESIAN_POINT('Ctrl Pts',(28.7938779355307,10.8625147335932,75.079826557824));
#49312=CARTESIAN_POINT('Ctrl Pts',(28.8019055096204,11.,75.1059958179575));
#49313=CARTESIAN_POINT('Ctrl Pts',(28.7938779355307,11.137485266407,75.079826557824));
#49314=CARTESIAN_POINT('Ctrl Pts',(28.7806136472154,11.2174765285995,75.0267085651774));
#49315=CARTESIAN_POINT('Ctrl Pts',(28.7683297787118,11.2789656668451,74.9656153280843));
#49316=CARTESIAN_POINT('Ctrl Pts',(28.7618133828337,11.3058394721478,74.9267618361903));
#49317=CARTESIAN_POINT('Ctrl Pts',(28.7525477553864,11.3414466364947,74.8410052800481));
#49318=CARTESIAN_POINT('Ctrl Pts',(28.7499717367413,11.3503212800739,74.7941254313177));
#49319=CARTESIAN_POINT('Ctrl Pts',(28.7499823739105,11.3502679248349,74.7059347785805));
#49320=CARTESIAN_POINT('Ctrl Pts',(28.7525231854577,11.3414465815878,74.65904064169));
#49321=CARTESIAN_POINT('Ctrl Pts',(28.7617930434695,11.3057060685816,74.5732868944695));
#49322=CARTESIAN_POINT('Ctrl Pts',(28.7683045654192,11.2788962751735,74.5344620266402));
#49323=CARTESIAN_POINT('Ctrl Pts',(28.7806043669257,11.2170846527409,74.4732883033298));
#49324=CARTESIAN_POINT('Ctrl Pts',(28.7871669871617,11.1779078402817,74.4468238161368));
#49325=CARTESIAN_POINT('Ctrl Pts',(28.7965453592084,11.0915510411579,74.4116063134345));
#49326=CARTESIAN_POINT('Ctrl Pts',(28.7991583057917,11.0443255072037,74.402898825339));
#49327=CARTESIAN_POINT('Ctrl Pts',(28.7991583057917,11.,74.402898825339));
#49328=CARTESIAN_POINT('Origin',(30.,11.,74.75));
#49329=CARTESIAN_POINT('',(31.1247090374087,11.0002124504859,75.0000451515836));
#49330=CARTESIAN_POINT('',(30.,11.,75.));
#49331=CARTESIAN_POINT('',(31.1247448713916,11.,74.5));
#49332=CARTESIAN_POINT('Ctrl Pts',(31.1247448713916,11.,74.5));
#49333=CARTESIAN_POINT('Ctrl Pts',(31.1247448713916,10.9659464908864,74.5));
#49334=CARTESIAN_POINT('Ctrl Pts',(31.1261756827447,10.9298345168618,74.5073000076697));
#49335=CARTESIAN_POINT('Ctrl Pts',(31.1339517690006,10.8327646136186,74.5515990517654));
#49336=CARTESIAN_POINT('Ctrl Pts',(31.1420908159051,10.7893390509663,74.6017232396597));
#49337=CARTESIAN_POINT('Ctrl Pts',(31.1476872898868,10.7609713644184,74.67535844061));
#49338=CARTESIAN_POINT('Ctrl Pts',(31.1494354031251,10.7527134717349,74.7054449809965));
#49339=CARTESIAN_POINT('Ctrl Pts',(31.1499942735367,10.7501398764272,74.7353946550602));
#49340=CARTESIAN_POINT('Ctrl Pts',(31.1500134121921,10.7500904271462,74.7788322674921));
#49341=CARTESIAN_POINT('Ctrl Pts',(31.1488155000854,10.7553567498143,74.8097236484711));
#49342=CARTESIAN_POINT('Ctrl Pts',(31.1443472815917,10.7777313954793,74.868459151291));
#49343=CARTESIAN_POINT('Ctrl Pts',(31.1411083085017,10.7951159561359,74.896430652982));
#49344=CARTESIAN_POINT('Ctrl Pts',(31.1347942340493,10.8375063649237,74.9423984737415));
#49345=CARTESIAN_POINT('Ctrl Pts',(31.127685335322,10.893977625089,74.984921689387));
#49346=CARTESIAN_POINT('Ctrl Pts',(31.1247224286309,10.9657107289254,74.9999918828307));
#49347=CARTESIAN_POINT('Ctrl Pts',(31.1247055431382,11.0002331671188,75.0000495544391));
#49348=CARTESIAN_POINT('Ctrl Pts',(31.1247055431382,11.0002331671188,75.0000495544391));
#49349=CARTESIAN_POINT('Ctrl Pts',(31.124701321765,11.0088637766672,75.0000639723411));
#49350=CARTESIAN_POINT('Ctrl Pts',(31.1250505782355,11.0430501864293,74.9982522876711));
#49351=CARTESIAN_POINT('Ctrl Pts',(31.1285913723511,11.1138410678152,74.9795740487944));
#49352=CARTESIAN_POINT('Ctrl Pts',(31.1347735960806,11.1625638434507,74.9425264014548));
#49353=CARTESIAN_POINT('Ctrl Pts',(31.1411018668555,11.2050979482099,74.8965372843256));
#49354=CARTESIAN_POINT('Ctrl Pts',(31.1443369970737,11.2224255640565,74.8685817070521));
#49355=CARTESIAN_POINT('Ctrl Pts',(31.1488131353229,11.2448334943903,74.8098480629189));
#49356=CARTESIAN_POINT('Ctrl Pts',(31.150002757725,11.2500769678483,74.7789675358608));
#49357=CARTESIAN_POINT('Ctrl Pts',(31.1500033272209,11.2500687651821,74.721048432782));
#49358=CARTESIAN_POINT('Ctrl Pts',(31.1488168576793,11.2448183482373,74.6901688043705));
#49359=CARTESIAN_POINT('Ctrl Pts',(31.1443391274454,11.2223904507778,74.6314330366943));
#49360=CARTESIAN_POINT('Ctrl Pts',(31.1411144986666,11.2050367965143,74.6034936013564));
#49361=CARTESIAN_POINT('Ctrl Pts',(31.1347817423216,11.1625707484721,74.5574686435559));
#49362=CARTESIAN_POINT('Ctrl Pts',(31.1312907402135,11.1345635586083,74.5363723884131));
#49363=CARTESIAN_POINT('Ctrl Pts',(31.1261983005099,11.0702714603723,74.5074842459491));
#49364=CARTESIAN_POINT('Ctrl Pts',(31.1247448713916,11.0340535091136,74.5));
#49365=CARTESIAN_POINT('Ctrl Pts',(31.1247448713916,11.,74.5));
#49366=CARTESIAN_POINT('Origin',(30.,0.0749999999999993,74.75));
#49367=CARTESIAN_POINT('',(30.,12.35,73.5));
#49368=CARTESIAN_POINT('Origin',(30.,12.35,74.75));
#49369=CARTESIAN_POINT('',(30.,-12.2,73.5));
#49370=CARTESIAN_POINT('',(30.,0.0749999999999993,73.5));
#49371=CARTESIAN_POINT('Origin',(30.,-12.2,74.75));
#49372=CARTESIAN_POINT('',(31.2008416942083,11.,74.402898825339));
#49373=CARTESIAN_POINT('Ctrl Pts',(31.2008416942083,11.,74.402898825339));
#49374=CARTESIAN_POINT('Ctrl Pts',(31.2008416942083,11.0443255072037,74.402898825339));
#49375=CARTESIAN_POINT('Ctrl Pts',(31.2034498953288,11.0915227449673,74.4115972952524));
#49376=CARTESIAN_POINT('Ctrl Pts',(31.2128253403987,11.177860265399,74.4468073082167));
#49377=CARTESIAN_POINT('Ctrl Pts',(31.219382667204,11.2170105083336,74.4732679137741));
#49378=CARTESIAN_POINT('Ctrl Pts',(31.2316840240808,11.2788159105534,74.5344263730226));
#49379=CARTESIAN_POINT('Ctrl Pts',(31.238178124029,11.3055670964467,74.5732631185048));
#49380=CARTESIAN_POINT('Ctrl Pts',(31.2474552469493,11.3412831677777,74.6590054383893));
#49381=CARTESIAN_POINT('Ctrl Pts',(31.2500082287207,11.3501163526545,74.7058957316331));
#49382=CARTESIAN_POINT('Ctrl Pts',(31.2500067841583,11.3501273161404,74.7940892347985));
#49383=CARTESIAN_POINT('Ctrl Pts',(31.2474485597635,11.3413050526674,74.8409763148676));
#49384=CARTESIAN_POINT('Ctrl Pts',(31.2381724030552,11.3056138390971,74.9267271045948));
#49385=CARTESIAN_POINT('Ctrl Pts',(31.2316599526739,11.2788954176252,74.9655685845438));
#49386=CARTESIAN_POINT('Ctrl Pts',(31.219366031553,11.2170074672431,75.0266815633276));
#49387=CARTESIAN_POINT('Ctrl Pts',(31.2077858172596,11.1489334478727,75.0729876097142));
#49388=CARTESIAN_POINT('Ctrl Pts',(31.2013950695966,11.0560522523136,75.0949726057065));
#49389=CARTESIAN_POINT('Ctrl Pts',(31.2001387800288,10.967068766035,75.099203566257));
#49390=CARTESIAN_POINT('Ctrl Pts',(31.2060936622365,10.8619583503284,75.0796341470907));
#49391=CARTESIAN_POINT('Ctrl Pts',(31.2193944389923,10.7831211214257,75.0265430631575));
#49392=CARTESIAN_POINT('Ctrl Pts',(31.231663625954,10.721424531713,74.9654333947178));
#49393=CARTESIAN_POINT('Ctrl Pts',(31.2381824498022,10.6946289834658,74.926572349275));
#49394=CARTESIAN_POINT('Ctrl Pts',(31.2474426701246,10.6589884763849,74.8408147269102));
#49395=CARTESIAN_POINT('Ctrl Pts',(31.2500188041202,10.6501203427759,74.7938953965327));
#49396=CARTESIAN_POINT('Ctrl Pts',(31.2499777517717,10.6502163880535,74.7277738109954));
#49397=CARTESIAN_POINT('Ctrl Pts',(31.2487735251553,10.6545117760602,74.6821698523604));
#49398=CARTESIAN_POINT('Ctrl Pts',(31.2451073934782,10.6679307949249,74.6374154183254));
#49399=CARTESIAN_POINT('Ctrl Pts',(31.2334589811991,10.7131771584539,74.5297226811336));
#49400=CARTESIAN_POINT('Ctrl Pts',(31.2176555102524,10.7784674980498,74.4652559194838));
#49401=CARTESIAN_POINT('Ctrl Pts',(31.2034310816527,10.9085549642993,74.4114322650177));
#49402=CARTESIAN_POINT('Ctrl Pts',(31.2008416942083,10.9556744927963,74.402898825339));
#49403=CARTESIAN_POINT('Ctrl Pts',(31.2008416942083,11.,74.402898825339));
#49404=CARTESIAN_POINT('Ctrl Pts',(31.2008416942083,11.,74.402898825339));
#49405=CARTESIAN_POINT('Ctrl Pts',(31.2008416942083,10.9556744927963,74.402898825339));
#49406=CARTESIAN_POINT('Ctrl Pts',(31.2034310816527,10.9085549642993,74.4114322650177));
#49407=CARTESIAN_POINT('Ctrl Pts',(31.2176555102524,10.7784674980498,74.4652559194838));
#49408=CARTESIAN_POINT('Ctrl Pts',(31.2334589811991,10.7131771584539,74.5297226811336));
#49409=CARTESIAN_POINT('Ctrl Pts',(31.2451073934782,10.6679307949249,74.6374154183254));
#49410=CARTESIAN_POINT('Ctrl Pts',(31.2487735251553,10.6545117760602,74.6821698523604));
#49411=CARTESIAN_POINT('Ctrl Pts',(31.2499777517717,10.6502163880535,74.7277738109954));
#49412=CARTESIAN_POINT('Ctrl Pts',(31.2500188041202,10.6501203427759,74.7938953965327));
#49413=CARTESIAN_POINT('Ctrl Pts',(31.2474426701246,10.6589884763849,74.8408147269102));
#49414=CARTESIAN_POINT('Ctrl Pts',(31.2381824498022,10.6946289834658,74.926572349275));
#49415=CARTESIAN_POINT('Ctrl Pts',(31.231663625954,10.721424531713,74.9654333947178));
#49416=CARTESIAN_POINT('Ctrl Pts',(31.2193944389923,10.7831211214257,75.0265430631575));
#49417=CARTESIAN_POINT('Ctrl Pts',(31.2060936622365,10.8619583503284,75.0796341470907));
#49418=CARTESIAN_POINT('Ctrl Pts',(31.2001387800288,10.967068766035,75.099203566257));
#49419=CARTESIAN_POINT('Ctrl Pts',(31.2013950695966,11.0560522523136,75.0949726057065));
#49420=CARTESIAN_POINT('Ctrl Pts',(31.2077858172596,11.1489334478727,75.0729876097142));
#49421=CARTESIAN_POINT('Ctrl Pts',(31.219366031553,11.2170074672431,75.0266815633276));
#49422=CARTESIAN_POINT('Ctrl Pts',(31.2316599526739,11.2788954176252,74.9655685845438));
#49423=CARTESIAN_POINT('Ctrl Pts',(31.2381724030552,11.3056138390971,74.9267271045948));
#49424=CARTESIAN_POINT('Ctrl Pts',(31.2474485597635,11.3413050526674,74.8409763148676));
#49425=CARTESIAN_POINT('Ctrl Pts',(31.2500067841583,11.3501273161404,74.7940892347985));
#49426=CARTESIAN_POINT('Ctrl Pts',(31.2500082287207,11.3501163526545,74.7058957316331));
#49427=CARTESIAN_POINT('Ctrl Pts',(31.2474552469493,11.3412831677777,74.6590054383893));
#49428=CARTESIAN_POINT('Ctrl Pts',(31.238178124029,11.3055670964467,74.5732631185048));
#49429=CARTESIAN_POINT('Ctrl Pts',(31.2316840240808,11.2788159105534,74.5344263730226));
#49430=CARTESIAN_POINT('Ctrl Pts',(31.219382667204,11.2170105083336,74.4732679137741));
#49431=CARTESIAN_POINT('Ctrl Pts',(31.2128253403987,11.177860265399,74.4468073082167));
#49432=CARTESIAN_POINT('Ctrl Pts',(31.2034498953288,11.0915227449673,74.4115972952524));
#49433=CARTESIAN_POINT('Ctrl Pts',(31.2008416942083,11.0443255072037,74.402898825339));
#49434=CARTESIAN_POINT('Ctrl Pts',(31.2008416942083,11.,74.402898825339));
#49435=CARTESIAN_POINT('Ctrl Pts',(31.1754760866027,11.,74.4352658835594));
#49436=CARTESIAN_POINT('Ctrl Pts',(31.1754825039498,10.9590934828951,74.4352569922628));
#49437=CARTESIAN_POINT('Ctrl Pts',(31.1776872705737,10.9156346775601,74.4434035072065));
#49438=CARTESIAN_POINT('Ctrl Pts',(31.1897460686789,10.7965923103755,74.4940126606344));
#49439=CARTESIAN_POINT('Ctrl Pts',(31.203023603427,10.7384950675313,74.5537875973164));
#49440=CARTESIAN_POINT('Ctrl Pts',(31.2126198620762,10.6990038501938,74.6500105505282));
#49441=CARTESIAN_POINT('Ctrl Pts',(31.2156609325165,10.6872473752913,74.6899269201168));
#49442=CARTESIAN_POINT('Ctrl Pts',(31.2166432344204,10.6835579773301,74.7302838024659));
#49443=CARTESIAN_POINT('Ctrl Pts',(31.2166789556008,10.6834636791878,74.7888557538772));
#49444=CARTESIAN_POINT('Ctrl Pts',(31.2145612377667,10.6911385284789,74.8304330234096));
#49445=CARTESIAN_POINT('Ctrl Pts',(31.2069013357892,10.7223471955558,74.9071783895744));
#49446=CARTESIAN_POINT('Ctrl Pts',(31.2014756711748,10.7460081723241,74.9424240072697));
#49447=CARTESIAN_POINT('Ctrl Pts',(31.1911904443518,10.8012679295396,74.9984625048355));
#49448=CARTESIAN_POINT('Ctrl Pts',(31.1799556567174,10.8726518369506,75.0480526205252));
#49449=CARTESIAN_POINT('Ctrl Pts',(31.174870941357,10.9696232075473,75.0667395509409));
#49450=CARTESIAN_POINT('Ctrl Pts',(31.1759381545625,11.0517459258799,75.0627103479815));
#49451=CARTESIAN_POINT('Ctrl Pts',(31.181383646221,11.1372451760654,75.0418355394467));
#49452=CARTESIAN_POINT('Ctrl Pts',(31.1911648504381,11.198886235768,74.9986042623894));
#49453=CARTESIAN_POINT('Ctrl Pts',(31.2014701628226,11.2542970310271,74.942558360535));
#49454=CARTESIAN_POINT('Ctrl Pts',(31.2068926720193,11.2779026324523,74.9073307299006));
#49455=CARTESIAN_POINT('Ctrl Pts',(31.2145655752016,11.3091504024221,74.8305998229589));
#49456=CARTESIAN_POINT('Ctrl Pts',(31.2166694778626,11.3167865617185,74.7890364518618));
#49457=CARTESIAN_POINT('Ctrl Pts',(31.216671810142,11.3167751295637,74.7109475137158));
#49458=CARTESIAN_POINT('Ctrl Pts',(31.2145709126828,11.3091292053491,74.6693866581129));
#49459=CARTESIAN_POINT('Ctrl Pts',(31.2069004985881,11.2778549144797,74.5926509937699));
#49460=CARTESIAN_POINT('Ctrl Pts',(31.2014913594011,11.2542241587106,74.5574480118848));
#49461=CARTESIAN_POINT('Ctrl Pts',(31.1911853119282,11.1988747330847,74.5013269976795));
#49462=CARTESIAN_POINT('Ctrl Pts',(31.1856476298239,11.163432158172,74.4766690551516));
#49463=CARTESIAN_POINT('Ctrl Pts',(31.1777005937812,11.0844410836489,74.4435491508169));
#49464=CARTESIAN_POINT('Ctrl Pts',(31.1754859791547,11.0409058106239,74.4352694871419));
#49465=CARTESIAN_POINT('Ctrl Pts',(31.1754760866027,11.,74.4352658835593));
#49466=CARTESIAN_POINT('Ctrl Pts',(31.1501104789971,11.,74.4676329417797));
#49467=CARTESIAN_POINT('Ctrl Pts',(31.15010406165,10.9625275007876,74.4676418330762));
#49468=CARTESIAN_POINT('Ctrl Pts',(31.1519194938237,10.922754803601,74.475328765481));
#49469=CARTESIAN_POINT('Ctrl Pts',(31.1618612105741,10.8146398012929,74.5228423106149));
#49470=CARTESIAN_POINT('Ctrl Pts',(31.1725261936772,10.7640211418889,74.5776583234768));
#49471=CARTESIAN_POINT('Ctrl Pts',(31.1801748212888,10.7298983091494,74.6627633084073));
#49472=CARTESIAN_POINT('Ctrl Pts',(31.1825479957639,10.7199778725037,74.6976879132401));
#49473=CARTESIAN_POINT('Ctrl Pts',(31.183328790888,10.7167982871505,74.7328846635897));
#49474=CARTESIAN_POINT('Ctrl Pts',(31.1833532607115,10.7167470907343,74.7838719101477));
#49475=CARTESIAN_POINT('Ctrl Pts',(31.1816969324434,10.7232066977203,74.8201053519717));
#49476=CARTESIAN_POINT('Ctrl Pts',(31.1756283956047,10.7500131833893,74.8878531109917));
#49477=CARTESIAN_POINT('Ctrl Pts',(31.1712962632809,10.7705323155248,74.9194400404301));
#49478=CARTESIAN_POINT('Ctrl Pts',(31.1629982286899,10.8193595568098,74.9704790320636));
#49479=CARTESIAN_POINT('Ctrl Pts',(31.1538233408412,10.8832841384667,75.0165032159526));
#49480=CARTESIAN_POINT('Ctrl Pts',(31.1496199039663,10.9721229253927,75.0343396723273));
#49481=CARTESIAN_POINT('Ctrl Pts',(31.1505074932696,11.047356512863,75.0305145453961));
#49482=CARTESIAN_POINT('Ctrl Pts',(31.1549935433897,11.1255293396224,75.010726119062));
#49483=CARTESIAN_POINT('Ctrl Pts',(31.1629747771955,11.1806850749257,74.9706037023929));
#49484=CARTESIAN_POINT('Ctrl Pts',(31.1712916567069,11.229696334808,74.9195475083345));
#49485=CARTESIAN_POINT('Ctrl Pts',(31.1756167281097,11.2501367707013,74.8879780817463));
#49486=CARTESIAN_POINT('Ctrl Pts',(31.1816961198849,11.2769881446356,74.8202245548277));
#49487=CARTESIAN_POINT('Ctrl Pts',(31.1833400640207,11.2834177222702,74.7840203187975));
#49488=CARTESIAN_POINT('Ctrl Pts',(31.1833397457996,11.2834099882729,74.7159966506994));
#49489=CARTESIAN_POINT('Ctrl Pts',(31.1817011919459,11.2769723106658,74.6797875846469));
#49490=CARTESIAN_POINT('Ctrl Pts',(31.1756167528863,11.2501026327447,74.6120451614292));
#49491=CARTESIAN_POINT('Ctrl Pts',(31.1713071633463,11.2296285483571,74.5804719624942));
#49492=CARTESIAN_POINT('Ctrl Pts',(31.1629790975973,11.1807065237209,74.5294095596505));
#49493=CARTESIAN_POINT('Ctrl Pts',(31.1584684507883,11.1489916658353,74.5065106414782));
#49494=CARTESIAN_POINT('Ctrl Pts',(31.1519476020576,11.0773531216907,74.4755323903846));
#49495=CARTESIAN_POINT('Ctrl Pts',(31.1501005864452,11.0374732056933,74.4676293381971));
#49496=CARTESIAN_POINT('Ctrl Pts',(31.1501104789971,11.,74.4676329417797));
#49497=CARTESIAN_POINT('Ctrl Pts',(31.1247448713916,11.,74.5));
#49498=CARTESIAN_POINT('Ctrl Pts',(31.1247448713916,10.9659464908864,74.5));
#49499=CARTESIAN_POINT('Ctrl Pts',(31.1261756827447,10.9298345168618,74.5073000076697));
#49500=CARTESIAN_POINT('Ctrl Pts',(31.1339517690006,10.8327646136186,74.5515990517654));
#49501=CARTESIAN_POINT('Ctrl Pts',(31.1420908159051,10.7893390509663,74.6017232396597));
#49502=CARTESIAN_POINT('Ctrl Pts',(31.1476872898868,10.7609713644184,74.67535844061));
#49503=CARTESIAN_POINT('Ctrl Pts',(31.1494354031251,10.7527134717349,74.7054449809965));
#49504=CARTESIAN_POINT('Ctrl Pts',(31.1499942735367,10.7501398764272,74.7353946550602));
#49505=CARTESIAN_POINT('Ctrl Pts',(31.1500134121921,10.7500904271462,74.7788322674921));
#49506=CARTESIAN_POINT('Ctrl Pts',(31.1488155000854,10.7553567498143,74.8097236484711));
#49507=CARTESIAN_POINT('Ctrl Pts',(31.1443472815917,10.7777313954793,74.868459151291));
#49508=CARTESIAN_POINT('Ctrl Pts',(31.1411083085017,10.7951159561359,74.896430652982));
#49509=CARTESIAN_POINT('Ctrl Pts',(31.1347942340493,10.8375063649237,74.9423984737415));
#49510=CARTESIAN_POINT('Ctrl Pts',(31.127685335322,10.893977625089,74.984921689387));
#49511=CARTESIAN_POINT('Ctrl Pts',(31.1243520652945,10.974677366905,75.0018756570112));
#49512=CARTESIAN_POINT('Ctrl Pts',(31.1250505782355,11.0430501864293,74.9982522876711));
#49513=CARTESIAN_POINT('Ctrl Pts',(31.1285913723511,11.1138410678152,74.9795740487944));
#49514=CARTESIAN_POINT('Ctrl Pts',(31.1347735960806,11.1625638434507,74.9425264014548));
#49515=CARTESIAN_POINT('Ctrl Pts',(31.1411018668555,11.2050979482099,74.8965372843256));
#49516=CARTESIAN_POINT('Ctrl Pts',(31.1443369970737,11.2224255640565,74.8685817070521));
#49517=CARTESIAN_POINT('Ctrl Pts',(31.1488131353229,11.2448334943903,74.8098480629189));
#49518=CARTESIAN_POINT('Ctrl Pts',(31.150002757725,11.2500769678483,74.7789675358608));
#49519=CARTESIAN_POINT('Ctrl Pts',(31.1500033272209,11.2500687651821,74.721048432782));
#49520=CARTESIAN_POINT('Ctrl Pts',(31.1488168576793,11.2448183482373,74.6901688043705));
#49521=CARTESIAN_POINT('Ctrl Pts',(31.1443391274454,11.2223904507778,74.6314330366943));
#49522=CARTESIAN_POINT('Ctrl Pts',(31.1411144986666,11.2050367965143,74.6034936013564));
#49523=CARTESIAN_POINT('Ctrl Pts',(31.1347817423216,11.1625707484721,74.5574686435559));
#49524=CARTESIAN_POINT('Ctrl Pts',(31.1312907402135,11.1345635586083,74.5363723884131));
#49525=CARTESIAN_POINT('Ctrl Pts',(31.1261983005099,11.0702714603723,74.5074842459491));
#49526=CARTESIAN_POINT('Ctrl Pts',(31.1247448713916,11.0340535091136,74.5));
#49527=CARTESIAN_POINT('Ctrl Pts',(31.1247448713916,11.,74.5));
#49528=CARTESIAN_POINT('',(31.2008416942083,11.,74.402898825339));
#49529=CARTESIAN_POINT('Origin',(30.,-13.6,72.55));
#49530=CARTESIAN_POINT('',(30.,-13.6,71.05));
#49531=CARTESIAN_POINT('Origin',(30.,-13.6,70.75));
#49532=CARTESIAN_POINT('Origin',(30.,-13.6,72.55));
#49533=CARTESIAN_POINT('',(29.5980419823739,-13.9,74.3045454545454));
#49534=CARTESIAN_POINT('',(30.,-13.82360679775,74.15));
#49535=CARTESIAN_POINT('Ctrl Pts',(29.5980419823739,-13.9,74.3045454545454));
#49536=CARTESIAN_POINT('Ctrl Pts',(29.6299329572115,-13.9,74.2757684824466));
#49537=CARTESIAN_POINT('Ctrl Pts',(29.6652052380112,-13.8937937433722,74.2501593480394));
#49538=CARTESIAN_POINT('Ctrl Pts',(29.7577242969844,-13.8709763234875,74.1975402590115));
#49539=CARTESIAN_POINT('Ctrl Pts',(29.8164159855257,-13.8512468382518,74.1753780693518));
#49540=CARTESIAN_POINT('Ctrl Pts',(29.9235631410305,-13.8279036783418,74.1530313303057));
#49541=CARTESIAN_POINT('Ctrl Pts',(29.9641370497313,-13.82360679775,74.15));
#49542=CARTESIAN_POINT('Ctrl Pts',(30.,-13.82360679775,74.15));
#49543=CARTESIAN_POINT('',(30.,-13.37639320225,74.15));
#49544=CARTESIAN_POINT('Ctrl Pts',(30.,-13.37639320225,74.15));
#49545=CARTESIAN_POINT('Ctrl Pts',(29.9794953753375,-13.37639320225,74.15));
#49546=CARTESIAN_POINT('Ctrl Pts',(29.9592909928131,-13.3750898546546,74.1510401268365));
#49547=CARTESIAN_POINT('Ctrl Pts',(29.8830224888261,-13.3659078861817,74.1588159892685));
#49548=CARTESIAN_POINT('Ctrl Pts',(29.8286898089983,-13.3504584038552,74.1723413828209));
#49549=CARTESIAN_POINT('Ctrl Pts',(29.7200329870219,-13.319457616754,74.2157256444075));
#49550=CARTESIAN_POINT('Ctrl Pts',(29.6643996251244,-13.3033848210483,74.2482102326836));
#49551=CARTESIAN_POINT('Ctrl Pts',(29.5791479058784,-13.298480523946,74.3199941647947));
#49552=CARTESIAN_POINT('Ctrl Pts',(29.5505013820635,-13.3029058495517,74.3506920895563));
#49553=CARTESIAN_POINT('Ctrl Pts',(29.5050267351839,-13.3246102878397,74.409048352129));
#49554=CARTESIAN_POINT('Ctrl Pts',(29.4870006484232,-13.3408915120094,74.4373454937145));
#49555=CARTESIAN_POINT('Ctrl Pts',(29.4588733912034,-13.3860723864243,74.4892250785234));
#49556=CARTESIAN_POINT('Ctrl Pts',(29.448875238238,-13.4134749329035,74.5120117456315));
#49557=CARTESIAN_POINT('Ctrl Pts',(29.4346676303895,-13.4777648036933,74.5480752194044));
#49558=CARTESIAN_POINT('Ctrl Pts',(29.4305259541235,-13.5139266743675,74.5609560195142));
#49559=CARTESIAN_POINT('Ctrl Pts',(29.4267888944086,-13.5902829562109,74.572614364528));
#49560=CARTESIAN_POINT('Ctrl Pts',(29.4270773491324,-13.6296654597012,74.5715559886456));
#49561=CARTESIAN_POINT('Ctrl Pts',(29.4326305328973,-13.7056202535665,74.554633868808));
#49562=CARTESIAN_POINT('Ctrl Pts',(29.4376557542476,-13.7415461681365,74.5395144153543));
#49563=CARTESIAN_POINT('Ctrl Pts',(29.4548984871125,-13.8038410670045,74.4983529291516));
#49564=CARTESIAN_POINT('Ctrl Pts',(29.466452665742,-13.8300026504726,74.4736261267548));
#49565=CARTESIAN_POINT('Ctrl Pts',(29.4978314302509,-13.8692698084774,74.4203192067732));
#49566=CARTESIAN_POINT('Ctrl Pts',(29.5162338339307,-13.8827010732779,74.3933136319637));
#49567=CARTESIAN_POINT('Ctrl Pts',(29.5568556753082,-13.8972216746017,74.3445242219706));
#49568=CARTESIAN_POINT('Ctrl Pts',(29.5766365525769,-13.9,74.3238607454443));
#49569=CARTESIAN_POINT('Ctrl Pts',(29.5980419823739,-13.9,74.3045454545454));
#49570=CARTESIAN_POINT('Ctrl Pts',(30.,-13.82360679775,74.15));
#49571=CARTESIAN_POINT('Ctrl Pts',(30.0139201627258,-13.82360679775,74.15));
#49572=CARTESIAN_POINT('Ctrl Pts',(30.0271307004912,-13.8242030380086,74.150481853825));
#49573=CARTESIAN_POINT('Ctrl Pts',(30.0951134270113,-13.8296487208663,74.1549872164826));
#49574=CARTESIAN_POINT('Ctrl Pts',(30.1470884450656,-13.8429898222123,74.1662249454546));
#49575=CARTESIAN_POINT('Ctrl Pts',(30.2564245659286,-13.8734934982371,74.2035250184848));
#49576=CARTESIAN_POINT('Ctrl Pts',(30.3181043027727,-13.8932621546788,74.236141432118));
#49577=CARTESIAN_POINT('Ctrl Pts',(30.4105948909293,-13.9020508296339,74.3100801712879));
#49578=CARTESIAN_POINT('Ctrl Pts',(30.4406865741523,-13.8991034314819,74.3408667023364));
#49579=CARTESIAN_POINT('Ctrl Pts',(30.4884374841349,-13.879935290849,74.3996958219046));
#49580=CARTESIAN_POINT('Ctrl Pts',(30.507427201871,-13.8649842245123,74.428279748768));
#49581=CARTESIAN_POINT('Ctrl Pts',(30.5373103969786,-13.8221497329062,74.4813585396897));
#49582=CARTESIAN_POINT('Ctrl Pts',(30.5480743028103,-13.7958333738599,74.5049645380456));
#49583=CARTESIAN_POINT('Ctrl Pts',(30.5635948407606,-13.7333355759204,74.5431596663098));
#49584=CARTESIAN_POINT('Ctrl Pts',(30.5682799532287,-13.6979191328649,74.5573393219793));
#49585=CARTESIAN_POINT('Ctrl Pts',(30.5730288490156,-13.6223329980383,74.5719664120908));
#49586=CARTESIAN_POINT('Ctrl Pts',(30.573190284946,-13.5829576742045,74.5724938084201));
#49587=CARTESIAN_POINT('Ctrl Pts',(30.5686945991741,-13.5063041854332,74.5585902148283));
#49588=CARTESIAN_POINT('Ctrl Pts',(30.5642619605433,-13.4697037615921,74.5448600382466));
#49589=CARTESIAN_POINT('Ctrl Pts',(30.5484494876966,-13.4053569359173,74.5058346202232));
#49590=CARTESIAN_POINT('Ctrl Pts',(30.5376532005426,-13.3778853487224,74.4817796353062));
#49591=CARTESIAN_POINT('Ctrl Pts',(30.5077927921875,-13.335976596918,74.4291088579952));
#49592=CARTESIAN_POINT('Ctrl Pts',(30.4901145600946,-13.3212359418054,74.4021046660281));
#49593=CARTESIAN_POINT('Ctrl Pts',(30.4463232765293,-13.3027154144527,74.3475057927709));
#49594=CARTESIAN_POINT('Ctrl Pts',(30.421280112191,-13.2991731666418,74.3211276524706));
#49595=CARTESIAN_POINT('Ctrl Pts',(30.3594460746035,-13.301324643572,74.2675478584065));
#49596=CARTESIAN_POINT('Ctrl Pts',(30.3225431038836,-13.308777580929,74.2420598906178));
#49597=CARTESIAN_POINT('Ctrl Pts',(30.2254396406629,-13.334067198621,74.1901817946429));
#49598=CARTESIAN_POINT('Ctrl Pts',(30.163336812327,-13.3549930609079,74.1688930877428));
#49599=CARTESIAN_POINT('Ctrl Pts',(30.0641239823376,-13.3732076629203,74.1524392990832));
#49600=CARTESIAN_POINT('Ctrl Pts',(30.0317030754474,-13.37639320225,74.15));
#49601=CARTESIAN_POINT('Ctrl Pts',(30.,-13.37639320225,74.15));
#49602=CARTESIAN_POINT('Origin',(30.,-13.525,74.75));
#49603=CARTESIAN_POINT('',(30.,-13.,74.15));
#49604=CARTESIAN_POINT('Origin',(30.,-13.,74.75));
#49605=CARTESIAN_POINT('',(30.,-13.525,74.15));
#49606=CARTESIAN_POINT('',(30.,-14.1,74.15));
#49607=CARTESIAN_POINT('',(30.,-13.525,74.15));
#49608=CARTESIAN_POINT('Origin',(30.,-14.1,74.75));
#49609=CARTESIAN_POINT('Origin',(30.,-14.2,75.25));
#49610=CARTESIAN_POINT('',(30.,-14.2,74.25));
#49611=CARTESIAN_POINT('Origin',(30.,-14.2,74.75));
#49612=CARTESIAN_POINT('Origin',(30.,-14.15,74.75));
#49613=CARTESIAN_POINT('',(30.,-14.15,74.2));
#49614=CARTESIAN_POINT('Origin',(30.,-13.,76.35));
#49615=CARTESIAN_POINT('',(30.,-13.,73.15));
#49616=CARTESIAN_POINT('Origin',(30.,-13.,74.75));
#49617=CARTESIAN_POINT('Origin',(30.,-12.95,74.75));
#49618=CARTESIAN_POINT('',(30.,-12.9,73.05));
#49619=CARTESIAN_POINT('Origin',(30.,-12.9,74.75));
#49620=CARTESIAN_POINT('',(30.,-12.95,73.1));
#49621=CARTESIAN_POINT('Origin',(30.,-12.6,74.75));
#49622=CARTESIAN_POINT('',(30.,-12.3,73.05));
#49623=CARTESIAN_POINT('Origin',(30.,-12.3,74.75));
#49624=CARTESIAN_POINT('',(30.,-12.6,73.05));
#49625=CARTESIAN_POINT('Origin',(30.,-12.25,74.75));
#49626=CARTESIAN_POINT('',(30.,-12.2,73.15));
#49627=CARTESIAN_POINT('Origin',(30.,-12.2,74.75));
#49628=CARTESIAN_POINT('',(30.,-12.25,73.1));
#49629=CARTESIAN_POINT('Origin',(30.,-12.2,76.));
#49630=CARTESIAN_POINT('Origin',(30.,12.425,74.75));
#49631=CARTESIAN_POINT('',(30.,12.5,73.65));
#49632=CARTESIAN_POINT('Origin',(30.,12.5,74.75));
#49633=CARTESIAN_POINT('',(30.,12.425,73.575));
#49634=CARTESIAN_POINT('Origin',(30.,12.5,74.75));
#71460=UNCERTAINTY_MEASURE_WITH_UNIT(LENGTH_MEASURE(0.001),#71493,
'DISTANCE_ACCURACY_VALUE',
'Maximum model space distance between geometric entities at asserted c
onnectivities');
#71471=UNCERTAINTY_MEASURE_WITH_UNIT(LENGTH_MEASURE(0.001),#71493,
'DISTANCE_ACCURACY_VALUE',
'Maximum model space distance between geometric entities at asserted c
onnectivities');
#71481=(
GEOMETRIC_REPRESENTATION_CONTEXT(3)
GLOBAL_UNCERTAINTY_ASSIGNED_CONTEXT((#71460))
GLOBAL_UNIT_ASSIGNED_CONTEXT((#71493,#71495,#71496))
REPRESENTATION_CONTEXT('','3D')
);
#71492=(
GEOMETRIC_REPRESENTATION_CONTEXT(3)
GLOBAL_UNCERTAINTY_ASSIGNED_CONTEXT((#71471))
GLOBAL_UNIT_ASSIGNED_CONTEXT((#71493,#71495,#71496))
REPRESENTATION_CONTEXT('','3D')
);
#71493=(
LENGTH_UNIT()
NAMED_UNIT(*)
SI_UNIT(.CENTI.,.METRE.)
);
#71495=(
NAMED_UNIT(*)
PLANE_ANGLE_UNIT()
SI_UNIT($,.RADIAN.)
);
#71496=(
NAMED_UNIT(*)
SI_UNIT($,.STERADIAN.)
SOLID_ANGLE_UNIT()
);
#71506=SHAPE_DEFINITION_REPRESENTATION(#71526,#71611);
#71526=PRODUCT_DEFINITION_SHAPE('',$,#71632);
#71611=SHAPE_REPRESENTATION('',(#29982),#71481);
#71622=PRODUCT_DEFINITION_CONTEXT('part definition',#71684,'design');
#71632=PRODUCT_DEFINITION('2026-10-19-03-21-53-578',
'05_Bed_Support_Pin_D25x255_Ring_Handle',#71652,#71622);
#71652=PRODUCT_DEFINITION_FORMATION('',$,#71695);
#71684=APPLICATION_CONTEXT(
'Core Data for Automotive Mechanical Design Process');
#71685=PRODUCT_CONTEXT('part definition',#71684,'mechanical');
#71695=PRODUCT('2026-10-19-03-21-53-578',
'05_Bed_Support_Pin_D25x255_Ring_Handle',$,(#71685));
#71881=COLOUR_RGB('Grey',0.48,0.52,0.57);
#71882=FILL_AREA_STYLE_COLOUR('',#71881);
#71883=FILL_AREA_STYLE('',(#71882));
#71884=SURFACE_STYLE_FILL_AREA(#71883);
#71885=SURFACE_SIDE_STYLE('',(#71884));
#71886=SURFACE_STYLE_USAGE(.BOTH.,#71885);
#71887=PRESENTATION_STYLE_ASSIGNMENT((#71886));
ENDSEC;
END-ISO-10303-21;
